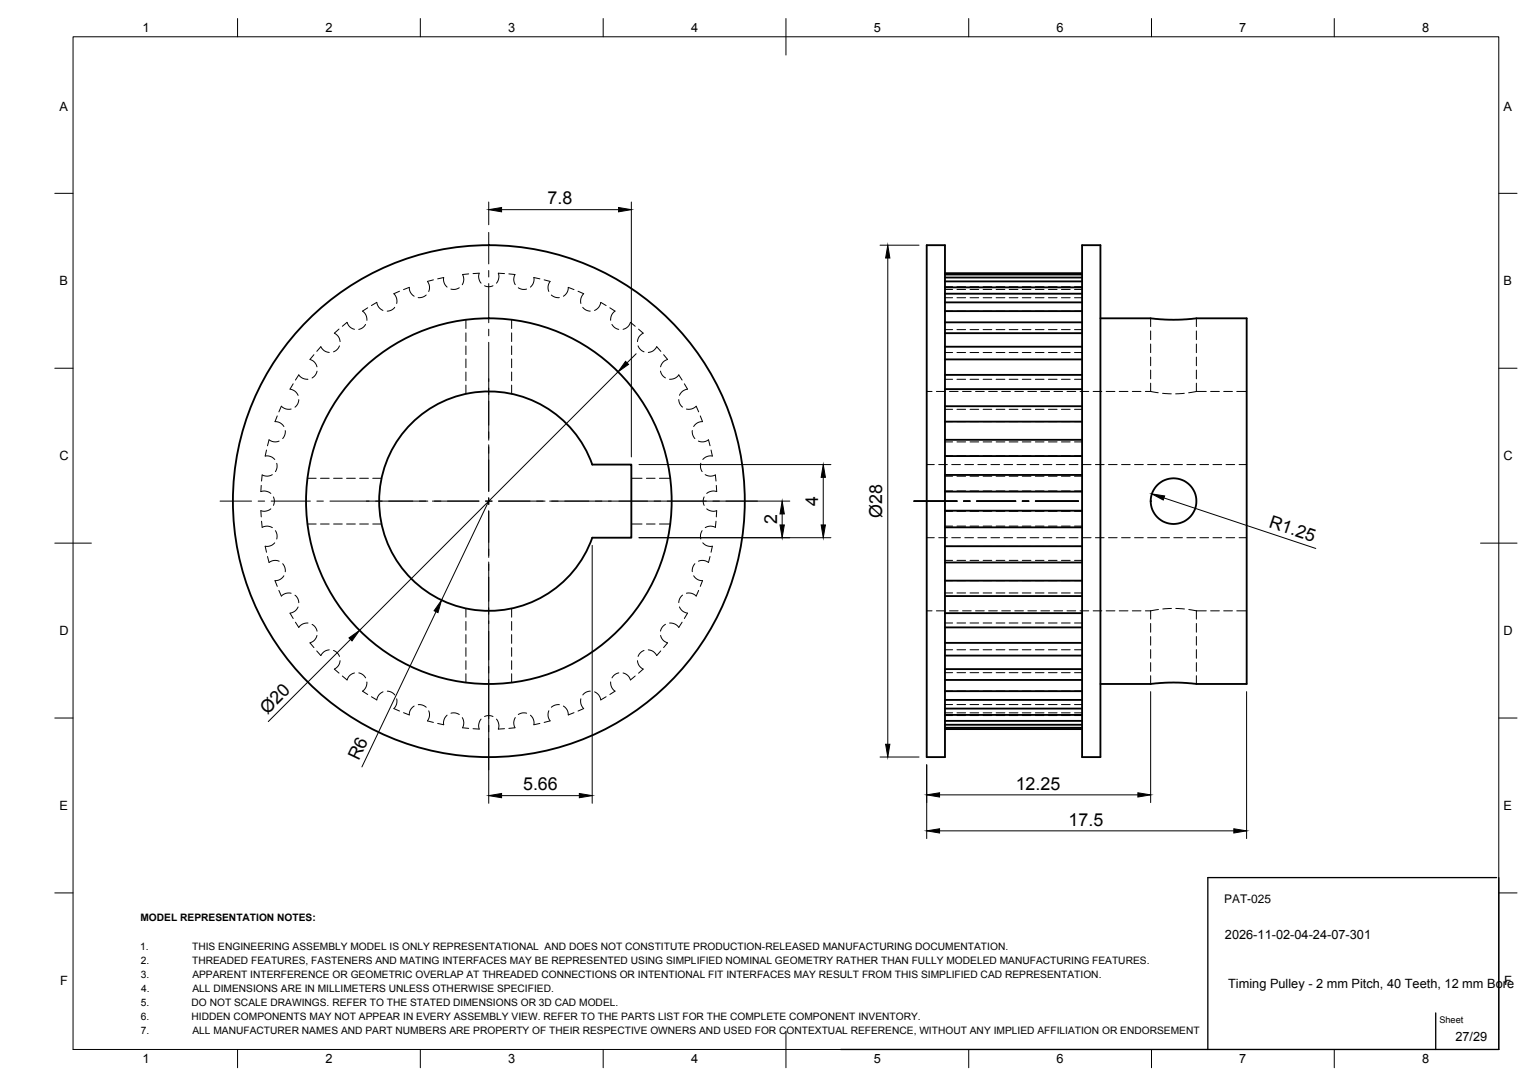
ISO-10303-21;
HEADER;
/* Generated by software containing ST-Developer
 * from STEP Tools, Inc. (www.steptools.com) 
 */

FILE_DESCRIPTION(
/* description */ ('Counter shaft with two pulleys and keyed hub'),
/* implementation_level */ '2;1');

FILE_NAME(
/* name */ 'Timing Pulley - 2 mm Pitch, 40 Teeth, 12 mm Bore.step',
/* time_stamp */ '2026-10-27T10:46:10-07:00',
/* author */ (''),
/* organization */ (''),
/* preprocessor_version */ 'ST-DEVELOPER v20.2',
/* originating_system */ 'Autodesk Translation Framework v15.17.0.0',
/* authorisation */ '');

FILE_SCHEMA (('AUTOMOTIVE_DESIGN { 1 0 10303 214 3 1 1 }'));
ENDSEC;

DATA;
#10=MECHANICAL_DESIGN_GEOMETRIC_PRESENTATION_REPRESENTATION('',(#311),#10821);
#220=B_SPLINE_CURVE_WITH_KNOTS('',3,(#9730,#9731,#9732,#9733,#9734,#9735,
#9736,#9737,#9738,#9739,#9740,#9741,#9742,#9743,#9744,#9745,#9746,#9747),
 .UNSPECIFIED.,.F.,.F.,(4,2,2,2,2,2,2,2,4),(0.,0.0472365751919841,0.0944731503839683,
0.14170659898184,0.188940047579712,0.236173496177583,0.283406944775455,
0.330643519967439,0.377880095159423),.UNSPECIFIED.);
#221=B_SPLINE_CURVE_WITH_KNOTS('',3,(#9748,#9749,#9750,#9751,#9752,#9753,
#9754,#9755,#9756,#9757,#9758,#9759,#9760,#9761,#9762,#9763,#9764,#9765),
 .UNSPECIFIED.,.F.,.F.,(4,2,2,2,2,2,2,2,4),(0.377880095159423,0.425116670351408,
0.472353245543392,0.519586694141263,0.566820142739135,0.614053591337007,
0.661287039934879,0.708523615126863,0.755760190318847),.UNSPECIFIED.);
#222=B_SPLINE_CURVE_WITH_KNOTS('',3,(#9768,#9769,#9770,#9771,#9772,#9773,
#9774,#9775,#9776,#9777,#9778,#9779,#9780,#9781,#9782,#9783,#9784,#9785),
 .UNSPECIFIED.,.F.,.F.,(4,2,2,2,2,2,2,2,4),(0.,0.0472365751919841,0.0944731503839682,
0.14170659898184,0.188940047579712,0.236173496177583,0.283406944775455,
0.330643519967439,0.377880095159423),.UNSPECIFIED.);
#223=B_SPLINE_CURVE_WITH_KNOTS('',3,(#9786,#9787,#9788,#9789,#9790,#9791,
#9792,#9793,#9794,#9795,#9796,#9797,#9798,#9799,#9800,#9801,#9802,#9803),
 .UNSPECIFIED.,.F.,.F.,(4,2,2,2,2,2,2,2,4),(0.377880095159423,0.425116670351408,
0.472353245543392,0.519586694141263,0.566820142739135,0.614053591337007,
0.661287039934879,0.708523615126863,0.755760190318847),.UNSPECIFIED.);
#224=B_SPLINE_CURVE_WITH_KNOTS('',3,(#9806,#9807,#9808,#9809,#9810,#9811,
#9812,#9813,#9814,#9815,#9816,#9817,#9818,#9819,#9820,#9821,#9822,#9823),
 .UNSPECIFIED.,.F.,.F.,(4,2,2,2,2,2,2,2,4),(0.,0.0472365751919841,0.0944731503839683,
0.14170659898184,0.188940047579712,0.236173496177583,0.283406944775455,
0.330643519967439,0.377880095159423),.UNSPECIFIED.);
#225=B_SPLINE_CURVE_WITH_KNOTS('',3,(#9824,#9825,#9826,#9827,#9828,#9829,
#9830,#9831,#9832,#9833,#9834,#9835,#9836,#9837,#9838,#9839,#9840,#9841),
 .UNSPECIFIED.,.F.,.F.,(4,2,2,2,2,2,2,2,4),(0.377880095159423,0.425116670351408,
0.472353245543392,0.519586694141263,0.566820142739135,0.614053591337007,
0.661287039934879,0.708523615126863,0.755760190318847),.UNSPECIFIED.);
#226=B_SPLINE_CURVE_WITH_KNOTS('',3,(#9845,#9846,#9847,#9848,#9849,#9850,
#9851,#9852,#9853,#9854),.UNSPECIFIED.,.F.,.F.,(4,2,2,2,4),(0.565665723963061,
0.61280433739166,0.659942950820258,0.70708195805217,0.754220965284082),
 .UNSPECIFIED.);
#227=B_SPLINE_CURVE_WITH_KNOTS('',3,(#9856,#9857,#9858,#9859,#9860,#9861,
#9862,#9863,#9864,#9865,#9866,#9867,#9868,#9869,#9870,#9871,#9872,#9873),
 .UNSPECIFIED.,.F.,.F.,(4,2,2,2,2,2,2,2,4),(0.18855524132102,0.235693854749619,
0.282832468178217,0.329971475410129,0.377110482642041,0.424249489873953,
0.471388497105864,0.518527110534463,0.565665723963061),.UNSPECIFIED.);
#228=B_SPLINE_CURVE_WITH_KNOTS('',3,(#9874,#9875,#9876,#9877,#9878,#9879,
#9880,#9881,#9882,#9883),.UNSPECIFIED.,.F.,.F.,(4,2,2,2,4),(0.754220965284082,
0.801359972515993,0.848498979747905,0.895637593176504,0.942776206605102),
 .UNSPECIFIED.);
#229=B_SPLINE_CURVE_WITH_KNOTS('',3,(#9889,#9890,#9891,#9892,#9893,#9894,
#9895,#9896,#9897,#9898),.UNSPECIFIED.,.F.,.F.,(4,2,2,2,4),(0.565665723963061,
0.61280433739166,0.659942950820258,0.70708195805217,0.754220965284082),
 .UNSPECIFIED.);
#230=B_SPLINE_CURVE_WITH_KNOTS('',3,(#9900,#9901,#9902,#9903,#9904,#9905,
#9906,#9907,#9908,#9909,#9910,#9911,#9912,#9913,#9914,#9915,#9916,#9917),
 .UNSPECIFIED.,.F.,.F.,(4,2,2,2,2,2,2,2,4),(0.18855524132102,0.235693854749619,
0.282832468178217,0.329971475410129,0.377110482642041,0.424249489873953,
0.471388497105864,0.518527110534463,0.565665723963061),.UNSPECIFIED.);
#231=B_SPLINE_CURVE_WITH_KNOTS('',3,(#9918,#9919,#9920,#9921,#9922,#9923,
#9924,#9925,#9926,#9927),.UNSPECIFIED.,.F.,.F.,(4,2,2,2,4),(0.754220965284082,
0.801359972515993,0.848498979747905,0.895637593176504,0.942776206605102),
 .UNSPECIFIED.);
#232=B_SPLINE_CURVE_WITH_KNOTS('',3,(#9937,#9938,#9939,#9940,#9941,#9942,
#9943,#9944,#9945,#9946,#9947,#9948,#9949,#9950,#9951,#9952,#9953,#9954),
 .UNSPECIFIED.,.F.,.F.,(4,2,2,2,2,2,2,2,4),(0.18855524132102,0.235693854749619,
0.282832468178217,0.329971475410129,0.377110482642041,0.424249489873953,
0.471388497105864,0.518527110534463,0.565665723963061),.UNSPECIFIED.);
#233=B_SPLINE_CURVE_WITH_KNOTS('',3,(#9956,#9957,#9958,#9959,#9960,#9961,
#9962,#9963,#9964,#9965),.UNSPECIFIED.,.F.,.F.,(4,2,2,2,4),(0.565665723963061,
0.61280433739166,0.659942950820258,0.70708195805217,0.754220965284082),
 .UNSPECIFIED.);
#234=B_SPLINE_CURVE_WITH_KNOTS('',3,(#9966,#9967,#9968,#9969,#9970,#9971,
#9972,#9973,#9974,#9975),.UNSPECIFIED.,.F.,.F.,(4,2,2,2,4),(0.754220965284082,
0.801359972515993,0.848498979747905,0.895637593176504,0.942776206605102),
 .UNSPECIFIED.);
#235=B_SPLINE_CURVE_WITH_KNOTS('',3,(#9978,#9979,#9980,#9981,#9982,#9983,
#9984,#9985,#9986,#9987,#9988,#9989,#9990,#9991,#9992,#9993,#9994,#9995),
 .UNSPECIFIED.,.F.,.F.,(4,2,2,2,2,2,2,2,4),(0.18855524132102,0.235693854749619,
0.282832468178217,0.329971475410129,0.377110482642041,0.424249489873953,
0.471388497105864,0.518527110534463,0.565665723963061),.UNSPECIFIED.);
#236=B_SPLINE_CURVE_WITH_KNOTS('',3,(#9997,#9998,#9999,#10000,#10001,#10002,
#10003,#10004,#10005,#10006),.UNSPECIFIED.,.F.,.F.,(4,2,2,2,4),(0.565665723963061,
0.61280433739166,0.659942950820258,0.70708195805217,0.754220965284082),
 .UNSPECIFIED.);
#237=B_SPLINE_CURVE_WITH_KNOTS('',3,(#10007,#10008,#10009,#10010,#10011,
#10012,#10013,#10014,#10015,#10016),.UNSPECIFIED.,.F.,.F.,(4,2,2,2,4),(0.754220965284082,
0.801359972515993,0.848498979747905,0.895637593176504,0.942776206605102),
 .UNSPECIFIED.);
#260=SHAPE_REPRESENTATION_RELATIONSHIP('SRR','None',#10948,#285);
#285=ADVANCED_BREP_SHAPE_REPRESENTATION('',(#336),#10816);
#311=STYLED_ITEM('',(#11128),#336);
#336=MANIFOLD_SOLID_BREP('Body1',#5595);
#417=FACE_BOUND('',#1150,.T.);
#418=FACE_BOUND('',#1153,.T.);
#419=FACE_BOUND('',#1155,.T.);
#420=FACE_BOUND('',#1156,.T.);
#421=FACE_BOUND('',#1157,.T.);
#422=FACE_BOUND('',#1161,.T.);
#423=FACE_BOUND('',#1162,.T.);
#424=FACE_BOUND('',#1163,.T.);
#425=FACE_BOUND('',#1167,.T.);
#426=FACE_BOUND('',#1169,.T.);
#427=FACE_BOUND('',#1172,.T.);
#428=FACE_BOUND('',#1174,.T.);
#540=PLANE('',#6208);
#541=PLANE('',#6209);
#542=PLANE('',#6211);
#543=PLANE('',#6212);
#544=PLANE('',#6224);
#545=PLANE('',#6225);
#546=PLANE('',#6309);
#547=PLANE('',#6310);
#757=FACE_OUTER_BOUND('',#1148,.T.);
#758=FACE_OUTER_BOUND('',#1149,.T.);
#759=FACE_OUTER_BOUND('',#1151,.T.);
#760=FACE_OUTER_BOUND('',#1152,.T.);
#761=FACE_OUTER_BOUND('',#1154,.T.);
#762=FACE_OUTER_BOUND('',#1158,.T.);
#763=FACE_OUTER_BOUND('',#1159,.T.);
#764=FACE_OUTER_BOUND('',#1160,.T.);
#765=FACE_OUTER_BOUND('',#1164,.T.);
#766=FACE_OUTER_BOUND('',#1165,.T.);
#767=FACE_OUTER_BOUND('',#1166,.T.);
#768=FACE_OUTER_BOUND('',#1168,.T.);
#769=FACE_OUTER_BOUND('',#1170,.T.);
#770=FACE_OUTER_BOUND('',#1171,.T.);
#771=FACE_OUTER_BOUND('',#1173,.T.);
#772=FACE_OUTER_BOUND('',#1175,.T.);
#773=FACE_OUTER_BOUND('',#1176,.T.);
#774=FACE_OUTER_BOUND('',#1177,.T.);
#775=FACE_OUTER_BOUND('',#1178,.T.);
#776=FACE_OUTER_BOUND('',#1179,.T.);
#777=FACE_OUTER_BOUND('',#1180,.T.);
#778=FACE_OUTER_BOUND('',#1181,.T.);
#779=FACE_OUTER_BOUND('',#1182,.T.);
#780=FACE_OUTER_BOUND('',#1183,.T.);
#781=FACE_OUTER_BOUND('',#1184,.T.);
#782=FACE_OUTER_BOUND('',#1185,.T.);
#783=FACE_OUTER_BOUND('',#1186,.T.);
#784=FACE_OUTER_BOUND('',#1187,.T.);
#785=FACE_OUTER_BOUND('',#1188,.T.);
#786=FACE_OUTER_BOUND('',#1189,.T.);
#787=FACE_OUTER_BOUND('',#1190,.T.);
#788=FACE_OUTER_BOUND('',#1191,.T.);
#789=FACE_OUTER_BOUND('',#1192,.T.);
#790=FACE_OUTER_BOUND('',#1193,.T.);
#791=FACE_OUTER_BOUND('',#1194,.T.);
#792=FACE_OUTER_BOUND('',#1195,.T.);
#793=FACE_OUTER_BOUND('',#1196,.T.);
#794=FACE_OUTER_BOUND('',#1197,.T.);
#795=FACE_OUTER_BOUND('',#1198,.T.);
#796=FACE_OUTER_BOUND('',#1199,.T.);
#797=FACE_OUTER_BOUND('',#1200,.T.);
#798=FACE_OUTER_BOUND('',#1201,.T.);
#799=FACE_OUTER_BOUND('',#1202,.T.);
#800=FACE_OUTER_BOUND('',#1203,.T.);
#801=FACE_OUTER_BOUND('',#1204,.T.);
#802=FACE_OUTER_BOUND('',#1205,.T.);
#803=FACE_OUTER_BOUND('',#1206,.T.);
#804=FACE_OUTER_BOUND('',#1207,.T.);
#805=FACE_OUTER_BOUND('',#1208,.T.);
#806=FACE_OUTER_BOUND('',#1209,.T.);
#807=FACE_OUTER_BOUND('',#1210,.T.);
#808=FACE_OUTER_BOUND('',#1211,.T.);
#809=FACE_OUTER_BOUND('',#1212,.T.);
#810=FACE_OUTER_BOUND('',#1213,.T.);
#811=FACE_OUTER_BOUND('',#1214,.T.);
#812=FACE_OUTER_BOUND('',#1215,.T.);
#813=FACE_OUTER_BOUND('',#1216,.T.);
#814=FACE_OUTER_BOUND('',#1217,.T.);
#815=FACE_OUTER_BOUND('',#1218,.T.);
#816=FACE_OUTER_BOUND('',#1219,.T.);
#817=FACE_OUTER_BOUND('',#1220,.T.);
#818=FACE_OUTER_BOUND('',#1221,.T.);
#819=FACE_OUTER_BOUND('',#1222,.T.);
#820=FACE_OUTER_BOUND('',#1223,.T.);
#821=FACE_OUTER_BOUND('',#1224,.T.);
#822=FACE_OUTER_BOUND('',#1225,.T.);
#823=FACE_OUTER_BOUND('',#1226,.T.);
#824=FACE_OUTER_BOUND('',#1227,.T.);
#825=FACE_OUTER_BOUND('',#1228,.T.);
#826=FACE_OUTER_BOUND('',#1229,.T.);
#827=FACE_OUTER_BOUND('',#1230,.T.);
#828=FACE_OUTER_BOUND('',#1231,.T.);
#829=FACE_OUTER_BOUND('',#1232,.T.);
#830=FACE_OUTER_BOUND('',#1233,.T.);
#831=FACE_OUTER_BOUND('',#1234,.T.);
#832=FACE_OUTER_BOUND('',#1235,.T.);
#833=FACE_OUTER_BOUND('',#1236,.T.);
#834=FACE_OUTER_BOUND('',#1237,.T.);
#835=FACE_OUTER_BOUND('',#1238,.T.);
#836=FACE_OUTER_BOUND('',#1239,.T.);
#837=FACE_OUTER_BOUND('',#1240,.T.);
#838=FACE_OUTER_BOUND('',#1241,.T.);
#839=FACE_OUTER_BOUND('',#1242,.T.);
#840=FACE_OUTER_BOUND('',#1243,.T.);
#841=FACE_OUTER_BOUND('',#1244,.T.);
#842=FACE_OUTER_BOUND('',#1245,.T.);
#843=FACE_OUTER_BOUND('',#1246,.T.);
#844=FACE_OUTER_BOUND('',#1247,.T.);
#845=FACE_OUTER_BOUND('',#1248,.T.);
#846=FACE_OUTER_BOUND('',#1249,.T.);
#847=FACE_OUTER_BOUND('',#1250,.T.);
#848=FACE_OUTER_BOUND('',#1251,.T.);
#849=FACE_OUTER_BOUND('',#1252,.T.);
#850=FACE_OUTER_BOUND('',#1253,.T.);
#851=FACE_OUTER_BOUND('',#1254,.T.);
#852=FACE_OUTER_BOUND('',#1255,.T.);
#1148=EDGE_LOOP('',(#4333,#4334,#4335,#4336));
#1149=EDGE_LOOP('',(#4337,#4338,#4339,#4340));
#1150=EDGE_LOOP('',(#4341));
#1151=EDGE_LOOP('',(#4342,#4343,#4344,#4345));
#1152=EDGE_LOOP('',(#4346));
#1153=EDGE_LOOP('',(#4347,#4348,#4349,#4350));
#1154=EDGE_LOOP('',(#4351,#4352,#4353,#4354));
#1155=EDGE_LOOP('',(#4355,#4356));
#1156=EDGE_LOOP('',(#4357,#4358));
#1157=EDGE_LOOP('',(#4359,#4360));
#1158=EDGE_LOOP('',(#4361,#4362,#4363,#4364,#4365,#4366,#4367));
#1159=EDGE_LOOP('',(#4368,#4369,#4370,#4371,#4372,#4373,#4374));
#1160=EDGE_LOOP('',(#4375,#4376,#4377,#4378,#4379,#4380,#4381,#4382,#4383));
#1161=EDGE_LOOP('',(#4384,#4385,#4386));
#1162=EDGE_LOOP('',(#4387,#4388,#4389));
#1163=EDGE_LOOP('',(#4390,#4391,#4392));
#1164=EDGE_LOOP('',(#4393,#4394,#4395,#4396,#4397,#4398));
#1165=EDGE_LOOP('',(#4399,#4400,#4401,#4402,#4403,#4404,#4405));
#1166=EDGE_LOOP('',(#4406));
#1167=EDGE_LOOP('',(#4407,#4408,#4409,#4410));
#1168=EDGE_LOOP('',(#4411));
#1169=EDGE_LOOP('',(#4412,#4413,#4414,#4415,#4416,#4417,#4418,#4419,#4420,
#4421,#4422,#4423,#4424,#4425,#4426,#4427,#4428,#4429,#4430,#4431,#4432,
#4433,#4434,#4435,#4436,#4437,#4438,#4439,#4440,#4441,#4442,#4443,#4444,
#4445,#4446,#4447,#4448,#4449,#4450,#4451,#4452,#4453,#4454,#4455,#4456,
#4457,#4458,#4459,#4460,#4461,#4462,#4463,#4464,#4465,#4466,#4467,#4468,
#4469,#4470,#4471,#4472,#4473,#4474,#4475,#4476,#4477,#4478,#4479,#4480,
#4481,#4482,#4483,#4484,#4485,#4486,#4487,#4488,#4489,#4490,#4491));
#1170=EDGE_LOOP('',(#4492,#4493,#4494,#4495));
#1171=EDGE_LOOP('',(#4496));
#1172=EDGE_LOOP('',(#4497));
#1173=EDGE_LOOP('',(#4498));
#1174=EDGE_LOOP('',(#4499,#4500,#4501,#4502,#4503,#4504,#4505,#4506,#4507,
#4508,#4509,#4510,#4511,#4512,#4513,#4514,#4515,#4516,#4517,#4518,#4519,
#4520,#4521,#4522,#4523,#4524,#4525,#4526,#4527,#4528,#4529,#4530,#4531,
#4532,#4533,#4534,#4535,#4536,#4537,#4538,#4539,#4540,#4541,#4542,#4543,
#4544,#4545,#4546,#4547,#4548,#4549,#4550,#4551,#4552,#4553,#4554,#4555,
#4556,#4557,#4558,#4559,#4560,#4561,#4562,#4563,#4564,#4565,#4566,#4567,
#4568,#4569,#4570,#4571,#4572,#4573,#4574,#4575,#4576,#4577,#4578));
#1175=EDGE_LOOP('',(#4579,#4580,#4581,#4582));
#1176=EDGE_LOOP('',(#4583,#4584,#4585,#4586));
#1177=EDGE_LOOP('',(#4587,#4588,#4589,#4590));
#1178=EDGE_LOOP('',(#4591,#4592,#4593,#4594));
#1179=EDGE_LOOP('',(#4595,#4596,#4597,#4598));
#1180=EDGE_LOOP('',(#4599,#4600,#4601,#4602));
#1181=EDGE_LOOP('',(#4603,#4604,#4605,#4606));
#1182=EDGE_LOOP('',(#4607,#4608,#4609,#4610));
#1183=EDGE_LOOP('',(#4611,#4612,#4613,#4614));
#1184=EDGE_LOOP('',(#4615,#4616,#4617,#4618));
#1185=EDGE_LOOP('',(#4619,#4620,#4621,#4622));
#1186=EDGE_LOOP('',(#4623,#4624,#4625,#4626));
#1187=EDGE_LOOP('',(#4627,#4628,#4629,#4630));
#1188=EDGE_LOOP('',(#4631,#4632,#4633,#4634));
#1189=EDGE_LOOP('',(#4635,#4636,#4637,#4638));
#1190=EDGE_LOOP('',(#4639,#4640,#4641,#4642));
#1191=EDGE_LOOP('',(#4643,#4644,#4645,#4646));
#1192=EDGE_LOOP('',(#4647,#4648,#4649,#4650));
#1193=EDGE_LOOP('',(#4651,#4652,#4653,#4654));
#1194=EDGE_LOOP('',(#4655,#4656,#4657,#4658));
#1195=EDGE_LOOP('',(#4659,#4660,#4661,#4662));
#1196=EDGE_LOOP('',(#4663,#4664,#4665,#4666));
#1197=EDGE_LOOP('',(#4667,#4668,#4669,#4670));
#1198=EDGE_LOOP('',(#4671,#4672,#4673,#4674));
#1199=EDGE_LOOP('',(#4675,#4676,#4677,#4678));
#1200=EDGE_LOOP('',(#4679,#4680,#4681,#4682));
#1201=EDGE_LOOP('',(#4683,#4684,#4685,#4686));
#1202=EDGE_LOOP('',(#4687,#4688,#4689,#4690));
#1203=EDGE_LOOP('',(#4691,#4692,#4693,#4694));
#1204=EDGE_LOOP('',(#4695,#4696,#4697,#4698));
#1205=EDGE_LOOP('',(#4699,#4700,#4701,#4702));
#1206=EDGE_LOOP('',(#4703,#4704,#4705,#4706));
#1207=EDGE_LOOP('',(#4707,#4708,#4709,#4710));
#1208=EDGE_LOOP('',(#4711,#4712,#4713,#4714));
#1209=EDGE_LOOP('',(#4715,#4716,#4717,#4718));
#1210=EDGE_LOOP('',(#4719,#4720,#4721,#4722));
#1211=EDGE_LOOP('',(#4723,#4724,#4725,#4726));
#1212=EDGE_LOOP('',(#4727,#4728,#4729,#4730));
#1213=EDGE_LOOP('',(#4731,#4732,#4733,#4734));
#1214=EDGE_LOOP('',(#4735,#4736,#4737,#4738));
#1215=EDGE_LOOP('',(#4739,#4740,#4741,#4742));
#1216=EDGE_LOOP('',(#4743,#4744,#4745,#4746));
#1217=EDGE_LOOP('',(#4747,#4748,#4749,#4750));
#1218=EDGE_LOOP('',(#4751,#4752,#4753,#4754));
#1219=EDGE_LOOP('',(#4755,#4756,#4757,#4758));
#1220=EDGE_LOOP('',(#4759,#4760,#4761,#4762));
#1221=EDGE_LOOP('',(#4763,#4764,#4765,#4766));
#1222=EDGE_LOOP('',(#4767,#4768,#4769,#4770));
#1223=EDGE_LOOP('',(#4771,#4772,#4773,#4774));
#1224=EDGE_LOOP('',(#4775,#4776,#4777,#4778));
#1225=EDGE_LOOP('',(#4779,#4780,#4781,#4782));
#1226=EDGE_LOOP('',(#4783,#4784,#4785,#4786));
#1227=EDGE_LOOP('',(#4787,#4788,#4789,#4790));
#1228=EDGE_LOOP('',(#4791,#4792,#4793,#4794));
#1229=EDGE_LOOP('',(#4795,#4796,#4797,#4798));
#1230=EDGE_LOOP('',(#4799,#4800,#4801,#4802));
#1231=EDGE_LOOP('',(#4803,#4804,#4805,#4806));
#1232=EDGE_LOOP('',(#4807,#4808,#4809,#4810));
#1233=EDGE_LOOP('',(#4811,#4812,#4813,#4814));
#1234=EDGE_LOOP('',(#4815,#4816,#4817,#4818));
#1235=EDGE_LOOP('',(#4819,#4820,#4821,#4822));
#1236=EDGE_LOOP('',(#4823,#4824,#4825,#4826));
#1237=EDGE_LOOP('',(#4827,#4828,#4829,#4830));
#1238=EDGE_LOOP('',(#4831,#4832,#4833,#4834));
#1239=EDGE_LOOP('',(#4835,#4836,#4837,#4838));
#1240=EDGE_LOOP('',(#4839,#4840,#4841,#4842));
#1241=EDGE_LOOP('',(#4843,#4844,#4845,#4846));
#1242=EDGE_LOOP('',(#4847,#4848,#4849,#4850));
#1243=EDGE_LOOP('',(#4851,#4852,#4853,#4854));
#1244=EDGE_LOOP('',(#4855,#4856,#4857,#4858));
#1245=EDGE_LOOP('',(#4859,#4860,#4861,#4862));
#1246=EDGE_LOOP('',(#4863,#4864,#4865,#4866));
#1247=EDGE_LOOP('',(#4867,#4868,#4869,#4870));
#1248=EDGE_LOOP('',(#4871,#4872,#4873,#4874));
#1249=EDGE_LOOP('',(#4875,#4876,#4877,#4878));
#1250=EDGE_LOOP('',(#4879,#4880,#4881,#4882));
#1251=EDGE_LOOP('',(#4883,#4884,#4885,#4886));
#1252=EDGE_LOOP('',(#4887,#4888,#4889,#4890));
#1253=EDGE_LOOP('',(#4891,#4892,#4893,#4894));
#1254=EDGE_LOOP('',(#4895,#4896,#4897,#4898));
#1255=EDGE_LOOP('',(#4899,#4900,#4901,#4902));
#1505=LINE('',#9702,#1894);
#1506=LINE('',#9704,#1895);
#1507=LINE('',#9706,#1896);
#1508=LINE('',#9707,#1897);
#1509=LINE('',#9710,#1898);
#1510=LINE('',#9712,#1899);
#1511=LINE('',#9713,#1900);
#1512=LINE('',#9718,#1901);
#1513=LINE('',#9720,#1902);
#1514=LINE('',#9721,#1903);
#1515=LINE('',#9884,#1904);
#1516=LINE('',#9887,#1905);
#1517=LINE('',#9931,#1906);
#1518=LINE('',#9933,#1907);
#1519=LINE('',#10018,#1908);
#1520=LINE('',#10020,#1909);
#1521=LINE('',#10188,#1910);
#1522=LINE('',#10354,#1911);
#1523=LINE('',#10356,#1912);
#1524=LINE('',#10357,#1913);
#1525=LINE('',#10359,#1914);
#1526=LINE('',#10361,#1915);
#1527=LINE('',#10363,#1916);
#1528=LINE('',#10365,#1917);
#1529=LINE('',#10367,#1918);
#1530=LINE('',#10369,#1919);
#1531=LINE('',#10371,#1920);
#1532=LINE('',#10373,#1921);
#1533=LINE('',#10375,#1922);
#1534=LINE('',#10377,#1923);
#1535=LINE('',#10379,#1924);
#1536=LINE('',#10381,#1925);
#1537=LINE('',#10383,#1926);
#1538=LINE('',#10385,#1927);
#1539=LINE('',#10387,#1928);
#1540=LINE('',#10389,#1929);
#1541=LINE('',#10391,#1930);
#1542=LINE('',#10393,#1931);
#1543=LINE('',#10395,#1932);
#1544=LINE('',#10397,#1933);
#1545=LINE('',#10399,#1934);
#1546=LINE('',#10401,#1935);
#1547=LINE('',#10403,#1936);
#1548=LINE('',#10405,#1937);
#1549=LINE('',#10407,#1938);
#1550=LINE('',#10409,#1939);
#1551=LINE('',#10411,#1940);
#1552=LINE('',#10413,#1941);
#1553=LINE('',#10415,#1942);
#1554=LINE('',#10417,#1943);
#1555=LINE('',#10419,#1944);
#1556=LINE('',#10421,#1945);
#1557=LINE('',#10423,#1946);
#1558=LINE('',#10425,#1947);
#1559=LINE('',#10427,#1948);
#1560=LINE('',#10429,#1949);
#1561=LINE('',#10431,#1950);
#1562=LINE('',#10433,#1951);
#1563=LINE('',#10435,#1952);
#1564=LINE('',#10437,#1953);
#1565=LINE('',#10439,#1954);
#1566=LINE('',#10441,#1955);
#1567=LINE('',#10443,#1956);
#1568=LINE('',#10445,#1957);
#1569=LINE('',#10447,#1958);
#1570=LINE('',#10449,#1959);
#1571=LINE('',#10451,#1960);
#1572=LINE('',#10453,#1961);
#1573=LINE('',#10455,#1962);
#1574=LINE('',#10457,#1963);
#1575=LINE('',#10459,#1964);
#1576=LINE('',#10461,#1965);
#1577=LINE('',#10463,#1966);
#1578=LINE('',#10465,#1967);
#1579=LINE('',#10467,#1968);
#1580=LINE('',#10469,#1969);
#1581=LINE('',#10471,#1970);
#1582=LINE('',#10473,#1971);
#1583=LINE('',#10475,#1972);
#1584=LINE('',#10477,#1973);
#1585=LINE('',#10479,#1974);
#1586=LINE('',#10481,#1975);
#1587=LINE('',#10483,#1976);
#1588=LINE('',#10485,#1977);
#1589=LINE('',#10487,#1978);
#1590=LINE('',#10489,#1979);
#1591=LINE('',#10491,#1980);
#1592=LINE('',#10493,#1981);
#1593=LINE('',#10495,#1982);
#1594=LINE('',#10497,#1983);
#1595=LINE('',#10499,#1984);
#1596=LINE('',#10501,#1985);
#1597=LINE('',#10503,#1986);
#1598=LINE('',#10505,#1987);
#1599=LINE('',#10507,#1988);
#1600=LINE('',#10509,#1989);
#1601=LINE('',#10511,#1990);
#1602=LINE('',#10513,#1991);
#1894=VECTOR('',#7421,1.);
#1895=VECTOR('',#7422,1.);
#1896=VECTOR('',#7423,1.);
#1897=VECTOR('',#7424,1.);
#1898=VECTOR('',#7427,1.);
#1899=VECTOR('',#7428,1.);
#1900=VECTOR('',#7429,1.);
#1901=VECTOR('',#7434,1.);
#1902=VECTOR('',#7435,1.);
#1903=VECTOR('',#7436,1.);
#1904=VECTOR('',#7449,0.125);
#1905=VECTOR('',#7452,0.125);
#1906=VECTOR('',#7457,1.);
#1907=VECTOR('',#7458,1.);
#1908=VECTOR('',#7463,0.125);
#1909=VECTOR('',#7466,0.125);
#1910=VECTOR('',#7637,1.4);
#1911=VECTOR('',#7806,1.4);
#1912=VECTOR('',#7809,1.);
#1913=VECTOR('',#7810,1.);
#1914=VECTOR('',#7813,1.);
#1915=VECTOR('',#7816,1.);
#1916=VECTOR('',#7819,1.);
#1917=VECTOR('',#7822,1.);
#1918=VECTOR('',#7825,1.);
#1919=VECTOR('',#7828,1.);
#1920=VECTOR('',#7831,1.);
#1921=VECTOR('',#7834,1.);
#1922=VECTOR('',#7837,1.);
#1923=VECTOR('',#7840,1.);
#1924=VECTOR('',#7843,1.);
#1925=VECTOR('',#7846,1.);
#1926=VECTOR('',#7849,1.);
#1927=VECTOR('',#7852,1.);
#1928=VECTOR('',#7855,1.);
#1929=VECTOR('',#7858,1.);
#1930=VECTOR('',#7861,1.);
#1931=VECTOR('',#7864,1.);
#1932=VECTOR('',#7867,1.);
#1933=VECTOR('',#7870,1.);
#1934=VECTOR('',#7873,1.);
#1935=VECTOR('',#7876,1.);
#1936=VECTOR('',#7879,1.);
#1937=VECTOR('',#7882,1.);
#1938=VECTOR('',#7885,1.);
#1939=VECTOR('',#7888,1.);
#1940=VECTOR('',#7891,1.);
#1941=VECTOR('',#7894,1.);
#1942=VECTOR('',#7897,1.);
#1943=VECTOR('',#7900,1.);
#1944=VECTOR('',#7903,1.);
#1945=VECTOR('',#7906,1.);
#1946=VECTOR('',#7909,1.);
#1947=VECTOR('',#7912,1.);
#1948=VECTOR('',#7915,1.);
#1949=VECTOR('',#7918,1.);
#1950=VECTOR('',#7921,1.);
#1951=VECTOR('',#7924,1.);
#1952=VECTOR('',#7927,1.);
#1953=VECTOR('',#7930,1.);
#1954=VECTOR('',#7933,1.);
#1955=VECTOR('',#7936,1.);
#1956=VECTOR('',#7939,1.);
#1957=VECTOR('',#7942,1.);
#1958=VECTOR('',#7945,1.);
#1959=VECTOR('',#7948,1.);
#1960=VECTOR('',#7951,1.);
#1961=VECTOR('',#7954,1.);
#1962=VECTOR('',#7957,1.);
#1963=VECTOR('',#7960,1.);
#1964=VECTOR('',#7963,1.);
#1965=VECTOR('',#7966,1.);
#1966=VECTOR('',#7969,1.);
#1967=VECTOR('',#7972,1.);
#1968=VECTOR('',#7975,1.);
#1969=VECTOR('',#7978,1.);
#1970=VECTOR('',#7981,1.);
#1971=VECTOR('',#7984,1.);
#1972=VECTOR('',#7987,1.);
#1973=VECTOR('',#7990,1.);
#1974=VECTOR('',#7993,1.);
#1975=VECTOR('',#7996,1.);
#1976=VECTOR('',#7999,1.);
#1977=VECTOR('',#8002,1.);
#1978=VECTOR('',#8005,1.);
#1979=VECTOR('',#8008,1.);
#1980=VECTOR('',#8011,1.);
#1981=VECTOR('',#8014,1.);
#1982=VECTOR('',#8017,1.);
#1983=VECTOR('',#8020,1.);
#1984=VECTOR('',#8023,1.);
#1985=VECTOR('',#8026,1.);
#1986=VECTOR('',#8029,1.);
#1987=VECTOR('',#8032,1.);
#1988=VECTOR('',#8035,1.);
#1989=VECTOR('',#8038,1.);
#1990=VECTOR('',#8041,1.);
#1991=VECTOR('',#8044,1.);
#2203=CIRCLE('',#6210,0.125);
#2204=CIRCLE('',#6213,1.4);
#2205=CIRCLE('',#6214,0.6);
#2206=CIRCLE('',#6216,0.6);
#2207=CIRCLE('',#6220,1.);
#2208=CIRCLE('',#6221,1.);
#2209=CIRCLE('',#6226,1.4);
#2210=CIRCLE('',#6227,0.0555000000000001);
#2211=CIRCLE('',#6228,1.24783954473516);
#2212=CIRCLE('',#6229,0.0555000000000001);
#2213=CIRCLE('',#6230,1.24783954473516);
#2214=CIRCLE('',#6231,0.0555000000000001);
#2215=CIRCLE('',#6232,1.24783954473516);
#2216=CIRCLE('',#6233,0.0555000000000001);
#2217=CIRCLE('',#6234,1.24783954473516);
#2218=CIRCLE('',#6235,0.0555000000000001);
#2219=CIRCLE('',#6236,1.24783954473516);
#2220=CIRCLE('',#6237,0.0555000000000001);
#2221=CIRCLE('',#6238,1.24783954473516);
#2222=CIRCLE('',#6239,0.0555000000000001);
#2223=CIRCLE('',#6240,1.24783954473516);
#2224=CIRCLE('',#6241,0.0555000000000001);
#2225=CIRCLE('',#6242,1.24783954473516);
#2226=CIRCLE('',#6243,0.0555000000000001);
#2227=CIRCLE('',#6244,1.24783954473516);
#2228=CIRCLE('',#6245,0.0555000000000001);
#2229=CIRCLE('',#6246,1.24783954473516);
#2230=CIRCLE('',#6247,0.0555000000000001);
#2231=CIRCLE('',#6248,1.24783954473516);
#2232=CIRCLE('',#6249,0.0555000000000001);
#2233=CIRCLE('',#6250,1.24783954473516);
#2234=CIRCLE('',#6251,0.0555000000000001);
#2235=CIRCLE('',#6252,1.24783954473516);
#2236=CIRCLE('',#6253,0.0555000000000001);
#2237=CIRCLE('',#6254,1.24783954473516);
#2238=CIRCLE('',#6255,0.0555000000000001);
#2239=CIRCLE('',#6256,1.24783954473516);
#2240=CIRCLE('',#6257,0.0555000000000001);
#2241=CIRCLE('',#6258,1.24783954473516);
#2242=CIRCLE('',#6259,0.0555000000000001);
#2243=CIRCLE('',#6260,1.24783954473516);
#2244=CIRCLE('',#6261,0.0555000000000001);
#2245=CIRCLE('',#6262,1.24783954473516);
#2246=CIRCLE('',#6263,0.0555000000000001);
#2247=CIRCLE('',#6264,1.24783954473516);
#2248=CIRCLE('',#6265,0.0555000000000001);
#2249=CIRCLE('',#6266,1.24783954473516);
#2250=CIRCLE('',#6267,0.0555000000000001);
#2251=CIRCLE('',#6268,1.24783954473516);
#2252=CIRCLE('',#6269,0.0555000000000001);
#2253=CIRCLE('',#6270,1.24783954473516);
#2254=CIRCLE('',#6271,0.0555000000000001);
#2255=CIRCLE('',#6272,1.24783954473516);
#2256=CIRCLE('',#6273,0.0555000000000001);
#2257=CIRCLE('',#6274,1.24783954473516);
#2258=CIRCLE('',#6275,0.0555000000000001);
#2259=CIRCLE('',#6276,1.24783954473516);
#2260=CIRCLE('',#6277,0.0555000000000001);
#2261=CIRCLE('',#6278,1.24783954473516);
#2262=CIRCLE('',#6279,0.0555000000000001);
#2263=CIRCLE('',#6280,1.24783954473516);
#2264=CIRCLE('',#6281,0.0555000000000001);
#2265=CIRCLE('',#6282,1.24783954473516);
#2266=CIRCLE('',#6283,0.0555000000000001);
#2267=CIRCLE('',#6284,1.24783954473516);
#2268=CIRCLE('',#6285,0.0555000000000001);
#2269=CIRCLE('',#6286,1.24783954473516);
#2270=CIRCLE('',#6287,0.0555000000000001);
#2271=CIRCLE('',#6288,1.24783954473516);
#2272=CIRCLE('',#6289,0.0555000000000001);
#2273=CIRCLE('',#6290,1.24783954473516);
#2274=CIRCLE('',#6291,0.0555000000000001);
#2275=CIRCLE('',#6292,1.24783954473516);
#2276=CIRCLE('',#6293,0.0555000000000001);
#2277=CIRCLE('',#6294,1.24783954473516);
#2278=CIRCLE('',#6295,0.0555000000000001);
#2279=CIRCLE('',#6296,1.24783954473516);
#2280=CIRCLE('',#6297,0.0555000000000001);
#2281=CIRCLE('',#6298,1.24783954473516);
#2282=CIRCLE('',#6299,0.0555000000000001);
#2283=CIRCLE('',#6300,1.24783954473516);
#2284=CIRCLE('',#6301,0.0555000000000001);
#2285=CIRCLE('',#6302,1.24783954473516);
#2286=CIRCLE('',#6303,0.0555000000000001);
#2287=CIRCLE('',#6304,1.24783954473516);
#2288=CIRCLE('',#6305,0.0555000000000001);
#2289=CIRCLE('',#6306,1.24783954473516);
#2290=CIRCLE('',#6308,1.4);
#2291=CIRCLE('',#6311,1.4);
#2292=CIRCLE('',#6312,0.0555000000000001);
#2293=CIRCLE('',#6313,1.24783954473516);
#2294=CIRCLE('',#6314,0.0555000000000001);
#2295=CIRCLE('',#6315,1.24783954473516);
#2296=CIRCLE('',#6316,0.0555000000000001);
#2297=CIRCLE('',#6317,1.24783954473516);
#2298=CIRCLE('',#6318,0.0555000000000001);
#2299=CIRCLE('',#6319,1.24783954473516);
#2300=CIRCLE('',#6320,0.0555000000000001);
#2301=CIRCLE('',#6321,1.24783954473516);
#2302=CIRCLE('',#6322,0.0555000000000001);
#2303=CIRCLE('',#6323,1.24783954473516);
#2304=CIRCLE('',#6324,0.0555000000000001);
#2305=CIRCLE('',#6325,1.24783954473516);
#2306=CIRCLE('',#6326,0.0555000000000001);
#2307=CIRCLE('',#6327,1.24783954473516);
#2308=CIRCLE('',#6328,0.0555000000000001);
#2309=CIRCLE('',#6329,1.24783954473516);
#2310=CIRCLE('',#6330,0.0555000000000001);
#2311=CIRCLE('',#6331,1.24783954473516);
#2312=CIRCLE('',#6332,0.0555000000000001);
#2313=CIRCLE('',#6333,1.24783954473516);
#2314=CIRCLE('',#6334,0.0555000000000001);
#2315=CIRCLE('',#6335,1.24783954473516);
#2316=CIRCLE('',#6336,0.0555000000000001);
#2317=CIRCLE('',#6337,1.24783954473516);
#2318=CIRCLE('',#6338,0.0555000000000001);
#2319=CIRCLE('',#6339,1.24783954473516);
#2320=CIRCLE('',#6340,0.0555000000000001);
#2321=CIRCLE('',#6341,1.24783954473516);
#2322=CIRCLE('',#6342,0.0555000000000001);
#2323=CIRCLE('',#6343,1.24783954473516);
#2324=CIRCLE('',#6344,0.0555000000000001);
#2325=CIRCLE('',#6345,1.24783954473516);
#2326=CIRCLE('',#6346,0.0555000000000001);
#2327=CIRCLE('',#6347,1.24783954473516);
#2328=CIRCLE('',#6348,0.0555000000000001);
#2329=CIRCLE('',#6349,1.24783954473516);
#2330=CIRCLE('',#6350,0.0555000000000001);
#2331=CIRCLE('',#6351,1.24783954473516);
#2332=CIRCLE('',#6352,0.0555000000000001);
#2333=CIRCLE('',#6353,1.24783954473516);
#2334=CIRCLE('',#6354,0.0555000000000001);
#2335=CIRCLE('',#6355,1.24783954473516);
#2336=CIRCLE('',#6356,0.0555000000000001);
#2337=CIRCLE('',#6357,1.24783954473516);
#2338=CIRCLE('',#6358,0.0555000000000001);
#2339=CIRCLE('',#6359,1.24783954473516);
#2340=CIRCLE('',#6360,0.0555000000000001);
#2341=CIRCLE('',#6361,1.24783954473516);
#2342=CIRCLE('',#6362,0.0555000000000001);
#2343=CIRCLE('',#6363,1.24783954473516);
#2344=CIRCLE('',#6364,0.0555000000000001);
#2345=CIRCLE('',#6365,1.24783954473516);
#2346=CIRCLE('',#6366,0.0555000000000001);
#2347=CIRCLE('',#6367,1.24783954473516);
#2348=CIRCLE('',#6368,0.0555000000000001);
#2349=CIRCLE('',#6369,1.24783954473516);
#2350=CIRCLE('',#6370,0.0555000000000001);
#2351=CIRCLE('',#6371,1.24783954473516);
#2352=CIRCLE('',#6372,0.0555000000000001);
#2353=CIRCLE('',#6373,1.24783954473516);
#2354=CIRCLE('',#6374,0.0555000000000001);
#2355=CIRCLE('',#6375,1.24783954473516);
#2356=CIRCLE('',#6376,0.0555000000000001);
#2357=CIRCLE('',#6377,1.24783954473516);
#2358=CIRCLE('',#6378,0.0555000000000001);
#2359=CIRCLE('',#6379,1.24783954473516);
#2360=CIRCLE('',#6380,0.0555000000000001);
#2361=CIRCLE('',#6381,1.24783954473516);
#2362=CIRCLE('',#6382,0.0555000000000001);
#2363=CIRCLE('',#6383,1.24783954473516);
#2364=CIRCLE('',#6384,0.0555000000000001);
#2365=CIRCLE('',#6385,1.24783954473516);
#2366=CIRCLE('',#6386,0.0555000000000001);
#2367=CIRCLE('',#6387,1.24783954473516);
#2368=CIRCLE('',#6388,0.0555000000000001);
#2369=CIRCLE('',#6389,1.24783954473516);
#2370=CIRCLE('',#6390,0.0555000000000001);
#2371=CIRCLE('',#6391,1.24783954473516);
#2626=VERTEX_POINT('',#9700);
#2627=VERTEX_POINT('',#9701);
#2628=VERTEX_POINT('',#9703);
#2629=VERTEX_POINT('',#9705);
#2630=VERTEX_POINT('',#9709);
#2631=VERTEX_POINT('',#9711);
#2632=VERTEX_POINT('',#9714);
#2633=VERTEX_POINT('',#9717);
#2634=VERTEX_POINT('',#9719);
#2635=VERTEX_POINT('',#9723);
#2636=VERTEX_POINT('',#9728);
#2637=VERTEX_POINT('',#9729);
#2638=VERTEX_POINT('',#9766);
#2639=VERTEX_POINT('',#9767);
#2640=VERTEX_POINT('',#9804);
#2641=VERTEX_POINT('',#9805);
#2642=VERTEX_POINT('',#9843);
#2643=VERTEX_POINT('',#9844);
#2644=VERTEX_POINT('',#9855);
#2645=VERTEX_POINT('',#9886);
#2646=VERTEX_POINT('',#9888);
#2647=VERTEX_POINT('',#9899);
#2648=VERTEX_POINT('',#9929);
#2649=VERTEX_POINT('',#9932);
#2650=VERTEX_POINT('',#9935);
#2651=VERTEX_POINT('',#9936);
#2652=VERTEX_POINT('',#9955);
#2653=VERTEX_POINT('',#9976);
#2654=VERTEX_POINT('',#9977);
#2655=VERTEX_POINT('',#9996);
#2656=VERTEX_POINT('',#10023);
#2657=VERTEX_POINT('',#10025);
#2658=VERTEX_POINT('',#10026);
#2659=VERTEX_POINT('',#10028);
#2660=VERTEX_POINT('',#10030);
#2661=VERTEX_POINT('',#10032);
#2662=VERTEX_POINT('',#10034);
#2663=VERTEX_POINT('',#10036);
#2664=VERTEX_POINT('',#10038);
#2665=VERTEX_POINT('',#10040);
#2666=VERTEX_POINT('',#10042);
#2667=VERTEX_POINT('',#10044);
#2668=VERTEX_POINT('',#10046);
#2669=VERTEX_POINT('',#10048);
#2670=VERTEX_POINT('',#10050);
#2671=VERTEX_POINT('',#10052);
#2672=VERTEX_POINT('',#10054);
#2673=VERTEX_POINT('',#10056);
#2674=VERTEX_POINT('',#10058);
#2675=VERTEX_POINT('',#10060);
#2676=VERTEX_POINT('',#10062);
#2677=VERTEX_POINT('',#10064);
#2678=VERTEX_POINT('',#10066);
#2679=VERTEX_POINT('',#10068);
#2680=VERTEX_POINT('',#10070);
#2681=VERTEX_POINT('',#10072);
#2682=VERTEX_POINT('',#10074);
#2683=VERTEX_POINT('',#10076);
#2684=VERTEX_POINT('',#10078);
#2685=VERTEX_POINT('',#10080);
#2686=VERTEX_POINT('',#10082);
#2687=VERTEX_POINT('',#10084);
#2688=VERTEX_POINT('',#10086);
#2689=VERTEX_POINT('',#10088);
#2690=VERTEX_POINT('',#10090);
#2691=VERTEX_POINT('',#10092);
#2692=VERTEX_POINT('',#10094);
#2693=VERTEX_POINT('',#10096);
#2694=VERTEX_POINT('',#10098);
#2695=VERTEX_POINT('',#10100);
#2696=VERTEX_POINT('',#10102);
#2697=VERTEX_POINT('',#10104);
#2698=VERTEX_POINT('',#10106);
#2699=VERTEX_POINT('',#10108);
#2700=VERTEX_POINT('',#10110);
#2701=VERTEX_POINT('',#10112);
#2702=VERTEX_POINT('',#10114);
#2703=VERTEX_POINT('',#10116);
#2704=VERTEX_POINT('',#10118);
#2705=VERTEX_POINT('',#10120);
#2706=VERTEX_POINT('',#10122);
#2707=VERTEX_POINT('',#10124);
#2708=VERTEX_POINT('',#10126);
#2709=VERTEX_POINT('',#10128);
#2710=VERTEX_POINT('',#10130);
#2711=VERTEX_POINT('',#10132);
#2712=VERTEX_POINT('',#10134);
#2713=VERTEX_POINT('',#10136);
#2714=VERTEX_POINT('',#10138);
#2715=VERTEX_POINT('',#10140);
#2716=VERTEX_POINT('',#10142);
#2717=VERTEX_POINT('',#10144);
#2718=VERTEX_POINT('',#10146);
#2719=VERTEX_POINT('',#10148);
#2720=VERTEX_POINT('',#10150);
#2721=VERTEX_POINT('',#10152);
#2722=VERTEX_POINT('',#10154);
#2723=VERTEX_POINT('',#10156);
#2724=VERTEX_POINT('',#10158);
#2725=VERTEX_POINT('',#10160);
#2726=VERTEX_POINT('',#10162);
#2727=VERTEX_POINT('',#10164);
#2728=VERTEX_POINT('',#10166);
#2729=VERTEX_POINT('',#10168);
#2730=VERTEX_POINT('',#10170);
#2731=VERTEX_POINT('',#10172);
#2732=VERTEX_POINT('',#10174);
#2733=VERTEX_POINT('',#10176);
#2734=VERTEX_POINT('',#10178);
#2735=VERTEX_POINT('',#10180);
#2736=VERTEX_POINT('',#10182);
#2737=VERTEX_POINT('',#10186);
#2738=VERTEX_POINT('',#10191);
#2739=VERTEX_POINT('',#10193);
#2740=VERTEX_POINT('',#10194);
#2741=VERTEX_POINT('',#10196);
#2742=VERTEX_POINT('',#10198);
#2743=VERTEX_POINT('',#10200);
#2744=VERTEX_POINT('',#10202);
#2745=VERTEX_POINT('',#10204);
#2746=VERTEX_POINT('',#10206);
#2747=VERTEX_POINT('',#10208);
#2748=VERTEX_POINT('',#10210);
#2749=VERTEX_POINT('',#10212);
#2750=VERTEX_POINT('',#10214);
#2751=VERTEX_POINT('',#10216);
#2752=VERTEX_POINT('',#10218);
#2753=VERTEX_POINT('',#10220);
#2754=VERTEX_POINT('',#10222);
#2755=VERTEX_POINT('',#10224);
#2756=VERTEX_POINT('',#10226);
#2757=VERTEX_POINT('',#10228);
#2758=VERTEX_POINT('',#10230);
#2759=VERTEX_POINT('',#10232);
#2760=VERTEX_POINT('',#10234);
#2761=VERTEX_POINT('',#10236);
#2762=VERTEX_POINT('',#10238);
#2763=VERTEX_POINT('',#10240);
#2764=VERTEX_POINT('',#10242);
#2765=VERTEX_POINT('',#10244);
#2766=VERTEX_POINT('',#10246);
#2767=VERTEX_POINT('',#10248);
#2768=VERTEX_POINT('',#10250);
#2769=VERTEX_POINT('',#10252);
#2770=VERTEX_POINT('',#10254);
#2771=VERTEX_POINT('',#10256);
#2772=VERTEX_POINT('',#10258);
#2773=VERTEX_POINT('',#10260);
#2774=VERTEX_POINT('',#10262);
#2775=VERTEX_POINT('',#10264);
#2776=VERTEX_POINT('',#10266);
#2777=VERTEX_POINT('',#10268);
#2778=VERTEX_POINT('',#10270);
#2779=VERTEX_POINT('',#10272);
#2780=VERTEX_POINT('',#10274);
#2781=VERTEX_POINT('',#10276);
#2782=VERTEX_POINT('',#10278);
#2783=VERTEX_POINT('',#10280);
#2784=VERTEX_POINT('',#10282);
#2785=VERTEX_POINT('',#10284);
#2786=VERTEX_POINT('',#10286);
#2787=VERTEX_POINT('',#10288);
#2788=VERTEX_POINT('',#10290);
#2789=VERTEX_POINT('',#10292);
#2790=VERTEX_POINT('',#10294);
#2791=VERTEX_POINT('',#10296);
#2792=VERTEX_POINT('',#10298);
#2793=VERTEX_POINT('',#10300);
#2794=VERTEX_POINT('',#10302);
#2795=VERTEX_POINT('',#10304);
#2796=VERTEX_POINT('',#10306);
#2797=VERTEX_POINT('',#10308);
#2798=VERTEX_POINT('',#10310);
#2799=VERTEX_POINT('',#10312);
#2800=VERTEX_POINT('',#10314);
#2801=VERTEX_POINT('',#10316);
#2802=VERTEX_POINT('',#10318);
#2803=VERTEX_POINT('',#10320);
#2804=VERTEX_POINT('',#10322);
#2805=VERTEX_POINT('',#10324);
#2806=VERTEX_POINT('',#10326);
#2807=VERTEX_POINT('',#10328);
#2808=VERTEX_POINT('',#10330);
#2809=VERTEX_POINT('',#10332);
#2810=VERTEX_POINT('',#10334);
#2811=VERTEX_POINT('',#10336);
#2812=VERTEX_POINT('',#10338);
#2813=VERTEX_POINT('',#10340);
#2814=VERTEX_POINT('',#10342);
#2815=VERTEX_POINT('',#10344);
#2816=VERTEX_POINT('',#10346);
#2817=VERTEX_POINT('',#10348);
#2818=VERTEX_POINT('',#10350);
#3239=EDGE_CURVE('',#2626,#2627,#1505,.T.);
#3240=EDGE_CURVE('',#2626,#2628,#1506,.T.);
#3241=EDGE_CURVE('',#2629,#2628,#1507,.T.);
#3242=EDGE_CURVE('',#2627,#2629,#1508,.T.);
#3243=EDGE_CURVE('',#2630,#2626,#1509,.T.);
#3244=EDGE_CURVE('',#2630,#2631,#1510,.T.);
#3245=EDGE_CURVE('',#2628,#2631,#1511,.T.);
#3246=EDGE_CURVE('',#2632,#2632,#2203,.T.);
#3247=EDGE_CURVE('',#2633,#2630,#1512,.T.);
#3248=EDGE_CURVE('',#2634,#2633,#1513,.T.);
#3249=EDGE_CURVE('',#2631,#2634,#1514,.T.);
#3250=EDGE_CURVE('',#2635,#2635,#2204,.T.);
#3251=EDGE_CURVE('',#2634,#2629,#2205,.T.);
#3252=EDGE_CURVE('',#2627,#2633,#2206,.T.);
#3253=EDGE_CURVE('',#2636,#2637,#220,.T.);
#3254=EDGE_CURVE('',#2637,#2636,#221,.T.);
#3255=EDGE_CURVE('',#2638,#2639,#222,.T.);
#3256=EDGE_CURVE('',#2639,#2638,#223,.T.);
#3257=EDGE_CURVE('',#2640,#2641,#224,.T.);
#3258=EDGE_CURVE('',#2641,#2640,#225,.T.);
#3259=EDGE_CURVE('',#2642,#2643,#226,.T.);
#3260=EDGE_CURVE('',#2644,#2642,#227,.T.);
#3261=EDGE_CURVE('',#2643,#2644,#228,.T.);
#3262=EDGE_CURVE('',#2643,#2639,#1515,.T.);
#3263=EDGE_CURVE('',#2641,#2645,#1516,.T.);
#3264=EDGE_CURVE('',#2646,#2645,#229,.T.);
#3265=EDGE_CURVE('',#2647,#2646,#230,.T.);
#3266=EDGE_CURVE('',#2645,#2647,#231,.T.);
#3267=EDGE_CURVE('',#2648,#2648,#2207,.T.);
#3268=EDGE_CURVE('',#2648,#2644,#1517,.T.);
#3269=EDGE_CURVE('',#2642,#2649,#1518,.T.);
#3270=EDGE_CURVE('',#2649,#2649,#2208,.T.);
#3271=EDGE_CURVE('',#2650,#2651,#232,.T.);
#3272=EDGE_CURVE('',#2651,#2652,#233,.T.);
#3273=EDGE_CURVE('',#2652,#2650,#234,.T.);
#3274=EDGE_CURVE('',#2653,#2654,#235,.T.);
#3275=EDGE_CURVE('',#2654,#2655,#236,.T.);
#3276=EDGE_CURVE('',#2655,#2653,#237,.T.);
#3277=EDGE_CURVE('',#2652,#2632,#1519,.T.);
#3278=EDGE_CURVE('',#2637,#2655,#1520,.T.);
#3279=EDGE_CURVE('',#2656,#2656,#2209,.T.);
#3280=EDGE_CURVE('',#2657,#2658,#2210,.T.);
#3281=EDGE_CURVE('',#2659,#2658,#2211,.T.);
#3282=EDGE_CURVE('',#2659,#2660,#2212,.T.);
#3283=EDGE_CURVE('',#2661,#2660,#2213,.T.);
#3284=EDGE_CURVE('',#2661,#2662,#2214,.T.);
#3285=EDGE_CURVE('',#2663,#2662,#2215,.T.);
#3286=EDGE_CURVE('',#2663,#2664,#2216,.T.);
#3287=EDGE_CURVE('',#2665,#2664,#2217,.T.);
#3288=EDGE_CURVE('',#2665,#2666,#2218,.T.);
#3289=EDGE_CURVE('',#2667,#2666,#2219,.T.);
#3290=EDGE_CURVE('',#2667,#2668,#2220,.T.);
#3291=EDGE_CURVE('',#2669,#2668,#2221,.T.);
#3292=EDGE_CURVE('',#2669,#2670,#2222,.T.);
#3293=EDGE_CURVE('',#2671,#2670,#2223,.T.);
#3294=EDGE_CURVE('',#2671,#2672,#2224,.T.);
#3295=EDGE_CURVE('',#2673,#2672,#2225,.T.);
#3296=EDGE_CURVE('',#2673,#2674,#2226,.T.);
#3297=EDGE_CURVE('',#2675,#2674,#2227,.T.);
#3298=EDGE_CURVE('',#2675,#2676,#2228,.T.);
#3299=EDGE_CURVE('',#2677,#2676,#2229,.T.);
#3300=EDGE_CURVE('',#2677,#2678,#2230,.T.);
#3301=EDGE_CURVE('',#2679,#2678,#2231,.T.);
#3302=EDGE_CURVE('',#2679,#2680,#2232,.T.);
#3303=EDGE_CURVE('',#2681,#2680,#2233,.T.);
#3304=EDGE_CURVE('',#2681,#2682,#2234,.T.);
#3305=EDGE_CURVE('',#2683,#2682,#2235,.T.);
#3306=EDGE_CURVE('',#2683,#2684,#2236,.T.);
#3307=EDGE_CURVE('',#2685,#2684,#2237,.T.);
#3308=EDGE_CURVE('',#2685,#2686,#2238,.T.);
#3309=EDGE_CURVE('',#2687,#2686,#2239,.T.);
#3310=EDGE_CURVE('',#2687,#2688,#2240,.T.);
#3311=EDGE_CURVE('',#2689,#2688,#2241,.T.);
#3312=EDGE_CURVE('',#2689,#2690,#2242,.T.);
#3313=EDGE_CURVE('',#2691,#2690,#2243,.T.);
#3314=EDGE_CURVE('',#2691,#2692,#2244,.T.);
#3315=EDGE_CURVE('',#2693,#2692,#2245,.T.);
#3316=EDGE_CURVE('',#2693,#2694,#2246,.T.);
#3317=EDGE_CURVE('',#2695,#2694,#2247,.T.);
#3318=EDGE_CURVE('',#2695,#2696,#2248,.T.);
#3319=EDGE_CURVE('',#2697,#2696,#2249,.T.);
#3320=EDGE_CURVE('',#2697,#2698,#2250,.T.);
#3321=EDGE_CURVE('',#2699,#2698,#2251,.T.);
#3322=EDGE_CURVE('',#2699,#2700,#2252,.T.);
#3323=EDGE_CURVE('',#2701,#2700,#2253,.T.);
#3324=EDGE_CURVE('',#2701,#2702,#2254,.T.);
#3325=EDGE_CURVE('',#2703,#2702,#2255,.T.);
#3326=EDGE_CURVE('',#2703,#2704,#2256,.T.);
#3327=EDGE_CURVE('',#2705,#2704,#2257,.T.);
#3328=EDGE_CURVE('',#2705,#2706,#2258,.T.);
#3329=EDGE_CURVE('',#2707,#2706,#2259,.T.);
#3330=EDGE_CURVE('',#2707,#2708,#2260,.T.);
#3331=EDGE_CURVE('',#2709,#2708,#2261,.T.);
#3332=EDGE_CURVE('',#2709,#2710,#2262,.T.);
#3333=EDGE_CURVE('',#2711,#2710,#2263,.T.);
#3334=EDGE_CURVE('',#2711,#2712,#2264,.T.);
#3335=EDGE_CURVE('',#2713,#2712,#2265,.T.);
#3336=EDGE_CURVE('',#2713,#2714,#2266,.T.);
#3337=EDGE_CURVE('',#2715,#2714,#2267,.T.);
#3338=EDGE_CURVE('',#2715,#2716,#2268,.T.);
#3339=EDGE_CURVE('',#2717,#2716,#2269,.T.);
#3340=EDGE_CURVE('',#2717,#2718,#2270,.T.);
#3341=EDGE_CURVE('',#2719,#2718,#2271,.T.);
#3342=EDGE_CURVE('',#2719,#2720,#2272,.T.);
#3343=EDGE_CURVE('',#2721,#2720,#2273,.T.);
#3344=EDGE_CURVE('',#2721,#2722,#2274,.T.);
#3345=EDGE_CURVE('',#2723,#2722,#2275,.T.);
#3346=EDGE_CURVE('',#2723,#2724,#2276,.T.);
#3347=EDGE_CURVE('',#2725,#2724,#2277,.T.);
#3348=EDGE_CURVE('',#2725,#2726,#2278,.T.);
#3349=EDGE_CURVE('',#2727,#2726,#2279,.T.);
#3350=EDGE_CURVE('',#2727,#2728,#2280,.T.);
#3351=EDGE_CURVE('',#2729,#2728,#2281,.T.);
#3352=EDGE_CURVE('',#2729,#2730,#2282,.T.);
#3353=EDGE_CURVE('',#2731,#2730,#2283,.T.);
#3354=EDGE_CURVE('',#2731,#2732,#2284,.T.);
#3355=EDGE_CURVE('',#2733,#2732,#2285,.T.);
#3356=EDGE_CURVE('',#2733,#2734,#2286,.T.);
#3357=EDGE_CURVE('',#2735,#2734,#2287,.T.);
#3358=EDGE_CURVE('',#2735,#2736,#2288,.T.);
#3359=EDGE_CURVE('',#2657,#2736,#2289,.T.);
#3360=EDGE_CURVE('',#2737,#2737,#2290,.T.);
#3361=EDGE_CURVE('',#2737,#2656,#1521,.T.);
#3362=EDGE_CURVE('',#2738,#2738,#2291,.T.);
#3363=EDGE_CURVE('',#2739,#2740,#2292,.T.);
#3364=EDGE_CURVE('',#2740,#2741,#2293,.T.);
#3365=EDGE_CURVE('',#2741,#2742,#2294,.T.);
#3366=EDGE_CURVE('',#2742,#2743,#2295,.T.);
#3367=EDGE_CURVE('',#2743,#2744,#2296,.T.);
#3368=EDGE_CURVE('',#2744,#2745,#2297,.T.);
#3369=EDGE_CURVE('',#2745,#2746,#2298,.T.);
#3370=EDGE_CURVE('',#2746,#2747,#2299,.T.);
#3371=EDGE_CURVE('',#2747,#2748,#2300,.T.);
#3372=EDGE_CURVE('',#2748,#2749,#2301,.T.);
#3373=EDGE_CURVE('',#2749,#2750,#2302,.T.);
#3374=EDGE_CURVE('',#2750,#2751,#2303,.T.);
#3375=EDGE_CURVE('',#2751,#2752,#2304,.T.);
#3376=EDGE_CURVE('',#2752,#2753,#2305,.T.);
#3377=EDGE_CURVE('',#2753,#2754,#2306,.T.);
#3378=EDGE_CURVE('',#2754,#2755,#2307,.T.);
#3379=EDGE_CURVE('',#2755,#2756,#2308,.T.);
#3380=EDGE_CURVE('',#2756,#2757,#2309,.T.);
#3381=EDGE_CURVE('',#2757,#2758,#2310,.T.);
#3382=EDGE_CURVE('',#2758,#2759,#2311,.T.);
#3383=EDGE_CURVE('',#2759,#2760,#2312,.T.);
#3384=EDGE_CURVE('',#2760,#2761,#2313,.T.);
#3385=EDGE_CURVE('',#2761,#2762,#2314,.T.);
#3386=EDGE_CURVE('',#2762,#2763,#2315,.T.);
#3387=EDGE_CURVE('',#2763,#2764,#2316,.T.);
#3388=EDGE_CURVE('',#2764,#2765,#2317,.T.);
#3389=EDGE_CURVE('',#2765,#2766,#2318,.T.);
#3390=EDGE_CURVE('',#2766,#2767,#2319,.T.);
#3391=EDGE_CURVE('',#2767,#2768,#2320,.T.);
#3392=EDGE_CURVE('',#2768,#2769,#2321,.T.);
#3393=EDGE_CURVE('',#2769,#2770,#2322,.T.);
#3394=EDGE_CURVE('',#2770,#2771,#2323,.T.);
#3395=EDGE_CURVE('',#2771,#2772,#2324,.T.);
#3396=EDGE_CURVE('',#2772,#2773,#2325,.T.);
#3397=EDGE_CURVE('',#2773,#2774,#2326,.T.);
#3398=EDGE_CURVE('',#2774,#2775,#2327,.T.);
#3399=EDGE_CURVE('',#2775,#2776,#2328,.T.);
#3400=EDGE_CURVE('',#2776,#2777,#2329,.T.);
#3401=EDGE_CURVE('',#2777,#2778,#2330,.T.);
#3402=EDGE_CURVE('',#2778,#2779,#2331,.T.);
#3403=EDGE_CURVE('',#2779,#2780,#2332,.T.);
#3404=EDGE_CURVE('',#2780,#2781,#2333,.T.);
#3405=EDGE_CURVE('',#2781,#2782,#2334,.T.);
#3406=EDGE_CURVE('',#2782,#2783,#2335,.T.);
#3407=EDGE_CURVE('',#2783,#2784,#2336,.T.);
#3408=EDGE_CURVE('',#2784,#2785,#2337,.T.);
#3409=EDGE_CURVE('',#2785,#2786,#2338,.T.);
#3410=EDGE_CURVE('',#2786,#2787,#2339,.T.);
#3411=EDGE_CURVE('',#2787,#2788,#2340,.T.);
#3412=EDGE_CURVE('',#2788,#2789,#2341,.T.);
#3413=EDGE_CURVE('',#2789,#2790,#2342,.T.);
#3414=EDGE_CURVE('',#2790,#2791,#2343,.T.);
#3415=EDGE_CURVE('',#2791,#2792,#2344,.T.);
#3416=EDGE_CURVE('',#2792,#2793,#2345,.T.);
#3417=EDGE_CURVE('',#2793,#2794,#2346,.T.);
#3418=EDGE_CURVE('',#2794,#2795,#2347,.T.);
#3419=EDGE_CURVE('',#2795,#2796,#2348,.T.);
#3420=EDGE_CURVE('',#2796,#2797,#2349,.T.);
#3421=EDGE_CURVE('',#2797,#2798,#2350,.T.);
#3422=EDGE_CURVE('',#2798,#2799,#2351,.T.);
#3423=EDGE_CURVE('',#2799,#2800,#2352,.T.);
#3424=EDGE_CURVE('',#2800,#2801,#2353,.T.);
#3425=EDGE_CURVE('',#2801,#2802,#2354,.T.);
#3426=EDGE_CURVE('',#2802,#2803,#2355,.T.);
#3427=EDGE_CURVE('',#2803,#2804,#2356,.T.);
#3428=EDGE_CURVE('',#2804,#2805,#2357,.T.);
#3429=EDGE_CURVE('',#2805,#2806,#2358,.T.);
#3430=EDGE_CURVE('',#2806,#2807,#2359,.T.);
#3431=EDGE_CURVE('',#2807,#2808,#2360,.T.);
#3432=EDGE_CURVE('',#2808,#2809,#2361,.T.);
#3433=EDGE_CURVE('',#2809,#2810,#2362,.T.);
#3434=EDGE_CURVE('',#2810,#2811,#2363,.T.);
#3435=EDGE_CURVE('',#2811,#2812,#2364,.T.);
#3436=EDGE_CURVE('',#2812,#2813,#2365,.T.);
#3437=EDGE_CURVE('',#2813,#2814,#2366,.T.);
#3438=EDGE_CURVE('',#2814,#2815,#2367,.T.);
#3439=EDGE_CURVE('',#2815,#2816,#2368,.T.);
#3440=EDGE_CURVE('',#2816,#2817,#2369,.T.);
#3441=EDGE_CURVE('',#2817,#2818,#2370,.T.);
#3442=EDGE_CURVE('',#2818,#2739,#2371,.T.);
#3443=EDGE_CURVE('',#2635,#2738,#1522,.T.);
#3444=EDGE_CURVE('',#2740,#2657,#1523,.T.);
#3445=EDGE_CURVE('',#2658,#2739,#1524,.T.);
#3446=EDGE_CURVE('',#2818,#2659,#1525,.T.);
#3447=EDGE_CURVE('',#2660,#2817,#1526,.T.);
#3448=EDGE_CURVE('',#2816,#2661,#1527,.T.);
#3449=EDGE_CURVE('',#2662,#2815,#1528,.T.);
#3450=EDGE_CURVE('',#2814,#2663,#1529,.T.);
#3451=EDGE_CURVE('',#2664,#2813,#1530,.T.);
#3452=EDGE_CURVE('',#2812,#2665,#1531,.T.);
#3453=EDGE_CURVE('',#2666,#2811,#1532,.T.);
#3454=EDGE_CURVE('',#2810,#2667,#1533,.T.);
#3455=EDGE_CURVE('',#2668,#2809,#1534,.T.);
#3456=EDGE_CURVE('',#2808,#2669,#1535,.T.);
#3457=EDGE_CURVE('',#2670,#2807,#1536,.T.);
#3458=EDGE_CURVE('',#2806,#2671,#1537,.T.);
#3459=EDGE_CURVE('',#2672,#2805,#1538,.T.);
#3460=EDGE_CURVE('',#2804,#2673,#1539,.T.);
#3461=EDGE_CURVE('',#2674,#2803,#1540,.T.);
#3462=EDGE_CURVE('',#2802,#2675,#1541,.T.);
#3463=EDGE_CURVE('',#2676,#2801,#1542,.T.);
#3464=EDGE_CURVE('',#2800,#2677,#1543,.T.);
#3465=EDGE_CURVE('',#2678,#2799,#1544,.T.);
#3466=EDGE_CURVE('',#2798,#2679,#1545,.T.);
#3467=EDGE_CURVE('',#2680,#2797,#1546,.T.);
#3468=EDGE_CURVE('',#2796,#2681,#1547,.T.);
#3469=EDGE_CURVE('',#2682,#2795,#1548,.T.);
#3470=EDGE_CURVE('',#2794,#2683,#1549,.T.);
#3471=EDGE_CURVE('',#2684,#2793,#1550,.T.);
#3472=EDGE_CURVE('',#2792,#2685,#1551,.T.);
#3473=EDGE_CURVE('',#2686,#2791,#1552,.T.);
#3474=EDGE_CURVE('',#2790,#2687,#1553,.T.);
#3475=EDGE_CURVE('',#2688,#2789,#1554,.T.);
#3476=EDGE_CURVE('',#2788,#2689,#1555,.T.);
#3477=EDGE_CURVE('',#2690,#2787,#1556,.T.);
#3478=EDGE_CURVE('',#2786,#2691,#1557,.T.);
#3479=EDGE_CURVE('',#2692,#2785,#1558,.T.);
#3480=EDGE_CURVE('',#2784,#2693,#1559,.T.);
#3481=EDGE_CURVE('',#2694,#2783,#1560,.T.);
#3482=EDGE_CURVE('',#2782,#2695,#1561,.T.);
#3483=EDGE_CURVE('',#2696,#2781,#1562,.T.);
#3484=EDGE_CURVE('',#2780,#2697,#1563,.T.);
#3485=EDGE_CURVE('',#2698,#2779,#1564,.T.);
#3486=EDGE_CURVE('',#2778,#2699,#1565,.T.);
#3487=EDGE_CURVE('',#2700,#2777,#1566,.T.);
#3488=EDGE_CURVE('',#2776,#2701,#1567,.T.);
#3489=EDGE_CURVE('',#2702,#2775,#1568,.T.);
#3490=EDGE_CURVE('',#2774,#2703,#1569,.T.);
#3491=EDGE_CURVE('',#2704,#2773,#1570,.T.);
#3492=EDGE_CURVE('',#2772,#2705,#1571,.T.);
#3493=EDGE_CURVE('',#2706,#2771,#1572,.T.);
#3494=EDGE_CURVE('',#2770,#2707,#1573,.T.);
#3495=EDGE_CURVE('',#2708,#2769,#1574,.T.);
#3496=EDGE_CURVE('',#2768,#2709,#1575,.T.);
#3497=EDGE_CURVE('',#2710,#2767,#1576,.T.);
#3498=EDGE_CURVE('',#2766,#2711,#1577,.T.);
#3499=EDGE_CURVE('',#2712,#2765,#1578,.T.);
#3500=EDGE_CURVE('',#2764,#2713,#1579,.T.);
#3501=EDGE_CURVE('',#2714,#2763,#1580,.T.);
#3502=EDGE_CURVE('',#2762,#2715,#1581,.T.);
#3503=EDGE_CURVE('',#2716,#2761,#1582,.T.);
#3504=EDGE_CURVE('',#2760,#2717,#1583,.T.);
#3505=EDGE_CURVE('',#2718,#2759,#1584,.T.);
#3506=EDGE_CURVE('',#2758,#2719,#1585,.T.);
#3507=EDGE_CURVE('',#2720,#2757,#1586,.T.);
#3508=EDGE_CURVE('',#2756,#2721,#1587,.T.);
#3509=EDGE_CURVE('',#2722,#2755,#1588,.T.);
#3510=EDGE_CURVE('',#2754,#2723,#1589,.T.);
#3511=EDGE_CURVE('',#2724,#2753,#1590,.T.);
#3512=EDGE_CURVE('',#2752,#2725,#1591,.T.);
#3513=EDGE_CURVE('',#2726,#2751,#1592,.T.);
#3514=EDGE_CURVE('',#2750,#2727,#1593,.T.);
#3515=EDGE_CURVE('',#2728,#2749,#1594,.T.);
#3516=EDGE_CURVE('',#2748,#2729,#1595,.T.);
#3517=EDGE_CURVE('',#2730,#2747,#1596,.T.);
#3518=EDGE_CURVE('',#2746,#2731,#1597,.T.);
#3519=EDGE_CURVE('',#2732,#2745,#1598,.T.);
#3520=EDGE_CURVE('',#2744,#2733,#1599,.T.);
#3521=EDGE_CURVE('',#2734,#2743,#1600,.T.);
#3522=EDGE_CURVE('',#2736,#2741,#1601,.T.);
#3523=EDGE_CURVE('',#2742,#2735,#1602,.T.);
#4333=ORIENTED_EDGE('',*,*,#3239,.F.);
#4334=ORIENTED_EDGE('',*,*,#3240,.T.);
#4335=ORIENTED_EDGE('',*,*,#3241,.F.);
#4336=ORIENTED_EDGE('',*,*,#3242,.F.);
#4337=ORIENTED_EDGE('',*,*,#3243,.F.);
#4338=ORIENTED_EDGE('',*,*,#3244,.T.);
#4339=ORIENTED_EDGE('',*,*,#3245,.F.);
#4340=ORIENTED_EDGE('',*,*,#3240,.F.);
#4341=ORIENTED_EDGE('',*,*,#3246,.F.);
#4342=ORIENTED_EDGE('',*,*,#3247,.F.);
#4343=ORIENTED_EDGE('',*,*,#3248,.F.);
#4344=ORIENTED_EDGE('',*,*,#3249,.F.);
#4345=ORIENTED_EDGE('',*,*,#3244,.F.);
#4346=ORIENTED_EDGE('',*,*,#3250,.T.);
#4347=ORIENTED_EDGE('',*,*,#3241,.T.);
#4348=ORIENTED_EDGE('',*,*,#3245,.T.);
#4349=ORIENTED_EDGE('',*,*,#3249,.T.);
#4350=ORIENTED_EDGE('',*,*,#3251,.T.);
#4351=ORIENTED_EDGE('',*,*,#3242,.T.);
#4352=ORIENTED_EDGE('',*,*,#3251,.F.);
#4353=ORIENTED_EDGE('',*,*,#3248,.T.);
#4354=ORIENTED_EDGE('',*,*,#3252,.F.);
#4355=ORIENTED_EDGE('',*,*,#3253,.T.);
#4356=ORIENTED_EDGE('',*,*,#3254,.T.);
#4357=ORIENTED_EDGE('',*,*,#3255,.T.);
#4358=ORIENTED_EDGE('',*,*,#3256,.T.);
#4359=ORIENTED_EDGE('',*,*,#3257,.T.);
#4360=ORIENTED_EDGE('',*,*,#3258,.T.);
#4361=ORIENTED_EDGE('',*,*,#3259,.F.);
#4362=ORIENTED_EDGE('',*,*,#3260,.F.);
#4363=ORIENTED_EDGE('',*,*,#3261,.F.);
#4364=ORIENTED_EDGE('',*,*,#3262,.T.);
#4365=ORIENTED_EDGE('',*,*,#3255,.F.);
#4366=ORIENTED_EDGE('',*,*,#3256,.F.);
#4367=ORIENTED_EDGE('',*,*,#3262,.F.);
#4368=ORIENTED_EDGE('',*,*,#3257,.F.);
#4369=ORIENTED_EDGE('',*,*,#3258,.F.);
#4370=ORIENTED_EDGE('',*,*,#3263,.T.);
#4371=ORIENTED_EDGE('',*,*,#3264,.F.);
#4372=ORIENTED_EDGE('',*,*,#3265,.F.);
#4373=ORIENTED_EDGE('',*,*,#3266,.F.);
#4374=ORIENTED_EDGE('',*,*,#3263,.F.);
#4375=ORIENTED_EDGE('',*,*,#3267,.F.);
#4376=ORIENTED_EDGE('',*,*,#3268,.T.);
#4377=ORIENTED_EDGE('',*,*,#3260,.T.);
#4378=ORIENTED_EDGE('',*,*,#3269,.T.);
#4379=ORIENTED_EDGE('',*,*,#3270,.F.);
#4380=ORIENTED_EDGE('',*,*,#3269,.F.);
#4381=ORIENTED_EDGE('',*,*,#3259,.T.);
#4382=ORIENTED_EDGE('',*,*,#3261,.T.);
#4383=ORIENTED_EDGE('',*,*,#3268,.F.);
#4384=ORIENTED_EDGE('',*,*,#3265,.T.);
#4385=ORIENTED_EDGE('',*,*,#3264,.T.);
#4386=ORIENTED_EDGE('',*,*,#3266,.T.);
#4387=ORIENTED_EDGE('',*,*,#3271,.T.);
#4388=ORIENTED_EDGE('',*,*,#3272,.T.);
#4389=ORIENTED_EDGE('',*,*,#3273,.T.);
#4390=ORIENTED_EDGE('',*,*,#3274,.T.);
#4391=ORIENTED_EDGE('',*,*,#3275,.T.);
#4392=ORIENTED_EDGE('',*,*,#3276,.T.);
#4393=ORIENTED_EDGE('',*,*,#3272,.F.);
#4394=ORIENTED_EDGE('',*,*,#3271,.F.);
#4395=ORIENTED_EDGE('',*,*,#3273,.F.);
#4396=ORIENTED_EDGE('',*,*,#3277,.T.);
#4397=ORIENTED_EDGE('',*,*,#3246,.T.);
#4398=ORIENTED_EDGE('',*,*,#3277,.F.);
#4399=ORIENTED_EDGE('',*,*,#3253,.F.);
#4400=ORIENTED_EDGE('',*,*,#3254,.F.);
#4401=ORIENTED_EDGE('',*,*,#3278,.T.);
#4402=ORIENTED_EDGE('',*,*,#3275,.F.);
#4403=ORIENTED_EDGE('',*,*,#3274,.F.);
#4404=ORIENTED_EDGE('',*,*,#3276,.F.);
#4405=ORIENTED_EDGE('',*,*,#3278,.F.);
#4406=ORIENTED_EDGE('',*,*,#3267,.T.);
#4407=ORIENTED_EDGE('',*,*,#3239,.T.);
#4408=ORIENTED_EDGE('',*,*,#3252,.T.);
#4409=ORIENTED_EDGE('',*,*,#3247,.T.);
#4410=ORIENTED_EDGE('',*,*,#3243,.T.);
#4411=ORIENTED_EDGE('',*,*,#3279,.T.);
#4412=ORIENTED_EDGE('',*,*,#3280,.T.);
#4413=ORIENTED_EDGE('',*,*,#3281,.F.);
#4414=ORIENTED_EDGE('',*,*,#3282,.T.);
#4415=ORIENTED_EDGE('',*,*,#3283,.F.);
#4416=ORIENTED_EDGE('',*,*,#3284,.T.);
#4417=ORIENTED_EDGE('',*,*,#3285,.F.);
#4418=ORIENTED_EDGE('',*,*,#3286,.T.);
#4419=ORIENTED_EDGE('',*,*,#3287,.F.);
#4420=ORIENTED_EDGE('',*,*,#3288,.T.);
#4421=ORIENTED_EDGE('',*,*,#3289,.F.);
#4422=ORIENTED_EDGE('',*,*,#3290,.T.);
#4423=ORIENTED_EDGE('',*,*,#3291,.F.);
#4424=ORIENTED_EDGE('',*,*,#3292,.T.);
#4425=ORIENTED_EDGE('',*,*,#3293,.F.);
#4426=ORIENTED_EDGE('',*,*,#3294,.T.);
#4427=ORIENTED_EDGE('',*,*,#3295,.F.);
#4428=ORIENTED_EDGE('',*,*,#3296,.T.);
#4429=ORIENTED_EDGE('',*,*,#3297,.F.);
#4430=ORIENTED_EDGE('',*,*,#3298,.T.);
#4431=ORIENTED_EDGE('',*,*,#3299,.F.);
#4432=ORIENTED_EDGE('',*,*,#3300,.T.);
#4433=ORIENTED_EDGE('',*,*,#3301,.F.);
#4434=ORIENTED_EDGE('',*,*,#3302,.T.);
#4435=ORIENTED_EDGE('',*,*,#3303,.F.);
#4436=ORIENTED_EDGE('',*,*,#3304,.T.);
#4437=ORIENTED_EDGE('',*,*,#3305,.F.);
#4438=ORIENTED_EDGE('',*,*,#3306,.T.);
#4439=ORIENTED_EDGE('',*,*,#3307,.F.);
#4440=ORIENTED_EDGE('',*,*,#3308,.T.);
#4441=ORIENTED_EDGE('',*,*,#3309,.F.);
#4442=ORIENTED_EDGE('',*,*,#3310,.T.);
#4443=ORIENTED_EDGE('',*,*,#3311,.F.);
#4444=ORIENTED_EDGE('',*,*,#3312,.T.);
#4445=ORIENTED_EDGE('',*,*,#3313,.F.);
#4446=ORIENTED_EDGE('',*,*,#3314,.T.);
#4447=ORIENTED_EDGE('',*,*,#3315,.F.);
#4448=ORIENTED_EDGE('',*,*,#3316,.T.);
#4449=ORIENTED_EDGE('',*,*,#3317,.F.);
#4450=ORIENTED_EDGE('',*,*,#3318,.T.);
#4451=ORIENTED_EDGE('',*,*,#3319,.F.);
#4452=ORIENTED_EDGE('',*,*,#3320,.T.);
#4453=ORIENTED_EDGE('',*,*,#3321,.F.);
#4454=ORIENTED_EDGE('',*,*,#3322,.T.);
#4455=ORIENTED_EDGE('',*,*,#3323,.F.);
#4456=ORIENTED_EDGE('',*,*,#3324,.T.);
#4457=ORIENTED_EDGE('',*,*,#3325,.F.);
#4458=ORIENTED_EDGE('',*,*,#3326,.T.);
#4459=ORIENTED_EDGE('',*,*,#3327,.F.);
#4460=ORIENTED_EDGE('',*,*,#3328,.T.);
#4461=ORIENTED_EDGE('',*,*,#3329,.F.);
#4462=ORIENTED_EDGE('',*,*,#3330,.T.);
#4463=ORIENTED_EDGE('',*,*,#3331,.F.);
#4464=ORIENTED_EDGE('',*,*,#3332,.T.);
#4465=ORIENTED_EDGE('',*,*,#3333,.F.);
#4466=ORIENTED_EDGE('',*,*,#3334,.T.);
#4467=ORIENTED_EDGE('',*,*,#3335,.F.);
#4468=ORIENTED_EDGE('',*,*,#3336,.T.);
#4469=ORIENTED_EDGE('',*,*,#3337,.F.);
#4470=ORIENTED_EDGE('',*,*,#3338,.T.);
#4471=ORIENTED_EDGE('',*,*,#3339,.F.);
#4472=ORIENTED_EDGE('',*,*,#3340,.T.);
#4473=ORIENTED_EDGE('',*,*,#3341,.F.);
#4474=ORIENTED_EDGE('',*,*,#3342,.T.);
#4475=ORIENTED_EDGE('',*,*,#3343,.F.);
#4476=ORIENTED_EDGE('',*,*,#3344,.T.);
#4477=ORIENTED_EDGE('',*,*,#3345,.F.);
#4478=ORIENTED_EDGE('',*,*,#3346,.T.);
#4479=ORIENTED_EDGE('',*,*,#3347,.F.);
#4480=ORIENTED_EDGE('',*,*,#3348,.T.);
#4481=ORIENTED_EDGE('',*,*,#3349,.F.);
#4482=ORIENTED_EDGE('',*,*,#3350,.T.);
#4483=ORIENTED_EDGE('',*,*,#3351,.F.);
#4484=ORIENTED_EDGE('',*,*,#3352,.T.);
#4485=ORIENTED_EDGE('',*,*,#3353,.F.);
#4486=ORIENTED_EDGE('',*,*,#3354,.T.);
#4487=ORIENTED_EDGE('',*,*,#3355,.F.);
#4488=ORIENTED_EDGE('',*,*,#3356,.T.);
#4489=ORIENTED_EDGE('',*,*,#3357,.F.);
#4490=ORIENTED_EDGE('',*,*,#3358,.T.);
#4491=ORIENTED_EDGE('',*,*,#3359,.F.);
#4492=ORIENTED_EDGE('',*,*,#3360,.F.);
#4493=ORIENTED_EDGE('',*,*,#3361,.T.);
#4494=ORIENTED_EDGE('',*,*,#3279,.F.);
#4495=ORIENTED_EDGE('',*,*,#3361,.F.);
#4496=ORIENTED_EDGE('',*,*,#3360,.T.);
#4497=ORIENTED_EDGE('',*,*,#3270,.T.);
#4498=ORIENTED_EDGE('',*,*,#3362,.F.);
#4499=ORIENTED_EDGE('',*,*,#3363,.T.);
#4500=ORIENTED_EDGE('',*,*,#3364,.T.);
#4501=ORIENTED_EDGE('',*,*,#3365,.T.);
#4502=ORIENTED_EDGE('',*,*,#3366,.T.);
#4503=ORIENTED_EDGE('',*,*,#3367,.T.);
#4504=ORIENTED_EDGE('',*,*,#3368,.T.);
#4505=ORIENTED_EDGE('',*,*,#3369,.T.);
#4506=ORIENTED_EDGE('',*,*,#3370,.T.);
#4507=ORIENTED_EDGE('',*,*,#3371,.T.);
#4508=ORIENTED_EDGE('',*,*,#3372,.T.);
#4509=ORIENTED_EDGE('',*,*,#3373,.T.);
#4510=ORIENTED_EDGE('',*,*,#3374,.T.);
#4511=ORIENTED_EDGE('',*,*,#3375,.T.);
#4512=ORIENTED_EDGE('',*,*,#3376,.T.);
#4513=ORIENTED_EDGE('',*,*,#3377,.T.);
#4514=ORIENTED_EDGE('',*,*,#3378,.T.);
#4515=ORIENTED_EDGE('',*,*,#3379,.T.);
#4516=ORIENTED_EDGE('',*,*,#3380,.T.);
#4517=ORIENTED_EDGE('',*,*,#3381,.T.);
#4518=ORIENTED_EDGE('',*,*,#3382,.T.);
#4519=ORIENTED_EDGE('',*,*,#3383,.T.);
#4520=ORIENTED_EDGE('',*,*,#3384,.T.);
#4521=ORIENTED_EDGE('',*,*,#3385,.T.);
#4522=ORIENTED_EDGE('',*,*,#3386,.T.);
#4523=ORIENTED_EDGE('',*,*,#3387,.T.);
#4524=ORIENTED_EDGE('',*,*,#3388,.T.);
#4525=ORIENTED_EDGE('',*,*,#3389,.T.);
#4526=ORIENTED_EDGE('',*,*,#3390,.T.);
#4527=ORIENTED_EDGE('',*,*,#3391,.T.);
#4528=ORIENTED_EDGE('',*,*,#3392,.T.);
#4529=ORIENTED_EDGE('',*,*,#3393,.T.);
#4530=ORIENTED_EDGE('',*,*,#3394,.T.);
#4531=ORIENTED_EDGE('',*,*,#3395,.T.);
#4532=ORIENTED_EDGE('',*,*,#3396,.T.);
#4533=ORIENTED_EDGE('',*,*,#3397,.T.);
#4534=ORIENTED_EDGE('',*,*,#3398,.T.);
#4535=ORIENTED_EDGE('',*,*,#3399,.T.);
#4536=ORIENTED_EDGE('',*,*,#3400,.T.);
#4537=ORIENTED_EDGE('',*,*,#3401,.T.);
#4538=ORIENTED_EDGE('',*,*,#3402,.T.);
#4539=ORIENTED_EDGE('',*,*,#3403,.T.);
#4540=ORIENTED_EDGE('',*,*,#3404,.T.);
#4541=ORIENTED_EDGE('',*,*,#3405,.T.);
#4542=ORIENTED_EDGE('',*,*,#3406,.T.);
#4543=ORIENTED_EDGE('',*,*,#3407,.T.);
#4544=ORIENTED_EDGE('',*,*,#3408,.T.);
#4545=ORIENTED_EDGE('',*,*,#3409,.T.);
#4546=ORIENTED_EDGE('',*,*,#3410,.T.);
#4547=ORIENTED_EDGE('',*,*,#3411,.T.);
#4548=ORIENTED_EDGE('',*,*,#3412,.T.);
#4549=ORIENTED_EDGE('',*,*,#3413,.T.);
#4550=ORIENTED_EDGE('',*,*,#3414,.T.);
#4551=ORIENTED_EDGE('',*,*,#3415,.T.);
#4552=ORIENTED_EDGE('',*,*,#3416,.T.);
#4553=ORIENTED_EDGE('',*,*,#3417,.T.);
#4554=ORIENTED_EDGE('',*,*,#3418,.T.);
#4555=ORIENTED_EDGE('',*,*,#3419,.T.);
#4556=ORIENTED_EDGE('',*,*,#3420,.T.);
#4557=ORIENTED_EDGE('',*,*,#3421,.T.);
#4558=ORIENTED_EDGE('',*,*,#3422,.T.);
#4559=ORIENTED_EDGE('',*,*,#3423,.T.);
#4560=ORIENTED_EDGE('',*,*,#3424,.T.);
#4561=ORIENTED_EDGE('',*,*,#3425,.T.);
#4562=ORIENTED_EDGE('',*,*,#3426,.T.);
#4563=ORIENTED_EDGE('',*,*,#3427,.T.);
#4564=ORIENTED_EDGE('',*,*,#3428,.T.);
#4565=ORIENTED_EDGE('',*,*,#3429,.T.);
#4566=ORIENTED_EDGE('',*,*,#3430,.T.);
#4567=ORIENTED_EDGE('',*,*,#3431,.T.);
#4568=ORIENTED_EDGE('',*,*,#3432,.T.);
#4569=ORIENTED_EDGE('',*,*,#3433,.T.);
#4570=ORIENTED_EDGE('',*,*,#3434,.T.);
#4571=ORIENTED_EDGE('',*,*,#3435,.T.);
#4572=ORIENTED_EDGE('',*,*,#3436,.T.);
#4573=ORIENTED_EDGE('',*,*,#3437,.T.);
#4574=ORIENTED_EDGE('',*,*,#3438,.T.);
#4575=ORIENTED_EDGE('',*,*,#3439,.T.);
#4576=ORIENTED_EDGE('',*,*,#3440,.T.);
#4577=ORIENTED_EDGE('',*,*,#3441,.T.);
#4578=ORIENTED_EDGE('',*,*,#3442,.T.);
#4579=ORIENTED_EDGE('',*,*,#3250,.F.);
#4580=ORIENTED_EDGE('',*,*,#3443,.T.);
#4581=ORIENTED_EDGE('',*,*,#3362,.T.);
#4582=ORIENTED_EDGE('',*,*,#3443,.F.);
#4583=ORIENTED_EDGE('',*,*,#3444,.F.);
#4584=ORIENTED_EDGE('',*,*,#3363,.F.);
#4585=ORIENTED_EDGE('',*,*,#3445,.F.);
#4586=ORIENTED_EDGE('',*,*,#3280,.F.);
#4587=ORIENTED_EDGE('',*,*,#3445,.T.);
#4588=ORIENTED_EDGE('',*,*,#3442,.F.);
#4589=ORIENTED_EDGE('',*,*,#3446,.T.);
#4590=ORIENTED_EDGE('',*,*,#3281,.T.);
#4591=ORIENTED_EDGE('',*,*,#3446,.F.);
#4592=ORIENTED_EDGE('',*,*,#3441,.F.);
#4593=ORIENTED_EDGE('',*,*,#3447,.F.);
#4594=ORIENTED_EDGE('',*,*,#3282,.F.);
#4595=ORIENTED_EDGE('',*,*,#3447,.T.);
#4596=ORIENTED_EDGE('',*,*,#3440,.F.);
#4597=ORIENTED_EDGE('',*,*,#3448,.T.);
#4598=ORIENTED_EDGE('',*,*,#3283,.T.);
#4599=ORIENTED_EDGE('',*,*,#3448,.F.);
#4600=ORIENTED_EDGE('',*,*,#3439,.F.);
#4601=ORIENTED_EDGE('',*,*,#3449,.F.);
#4602=ORIENTED_EDGE('',*,*,#3284,.F.);
#4603=ORIENTED_EDGE('',*,*,#3449,.T.);
#4604=ORIENTED_EDGE('',*,*,#3438,.F.);
#4605=ORIENTED_EDGE('',*,*,#3450,.T.);
#4606=ORIENTED_EDGE('',*,*,#3285,.T.);
#4607=ORIENTED_EDGE('',*,*,#3450,.F.);
#4608=ORIENTED_EDGE('',*,*,#3437,.F.);
#4609=ORIENTED_EDGE('',*,*,#3451,.F.);
#4610=ORIENTED_EDGE('',*,*,#3286,.F.);
#4611=ORIENTED_EDGE('',*,*,#3451,.T.);
#4612=ORIENTED_EDGE('',*,*,#3436,.F.);
#4613=ORIENTED_EDGE('',*,*,#3452,.T.);
#4614=ORIENTED_EDGE('',*,*,#3287,.T.);
#4615=ORIENTED_EDGE('',*,*,#3452,.F.);
#4616=ORIENTED_EDGE('',*,*,#3435,.F.);
#4617=ORIENTED_EDGE('',*,*,#3453,.F.);
#4618=ORIENTED_EDGE('',*,*,#3288,.F.);
#4619=ORIENTED_EDGE('',*,*,#3453,.T.);
#4620=ORIENTED_EDGE('',*,*,#3434,.F.);
#4621=ORIENTED_EDGE('',*,*,#3454,.T.);
#4622=ORIENTED_EDGE('',*,*,#3289,.T.);
#4623=ORIENTED_EDGE('',*,*,#3454,.F.);
#4624=ORIENTED_EDGE('',*,*,#3433,.F.);
#4625=ORIENTED_EDGE('',*,*,#3455,.F.);
#4626=ORIENTED_EDGE('',*,*,#3290,.F.);
#4627=ORIENTED_EDGE('',*,*,#3455,.T.);
#4628=ORIENTED_EDGE('',*,*,#3432,.F.);
#4629=ORIENTED_EDGE('',*,*,#3456,.T.);
#4630=ORIENTED_EDGE('',*,*,#3291,.T.);
#4631=ORIENTED_EDGE('',*,*,#3456,.F.);
#4632=ORIENTED_EDGE('',*,*,#3431,.F.);
#4633=ORIENTED_EDGE('',*,*,#3457,.F.);
#4634=ORIENTED_EDGE('',*,*,#3292,.F.);
#4635=ORIENTED_EDGE('',*,*,#3457,.T.);
#4636=ORIENTED_EDGE('',*,*,#3430,.F.);
#4637=ORIENTED_EDGE('',*,*,#3458,.T.);
#4638=ORIENTED_EDGE('',*,*,#3293,.T.);
#4639=ORIENTED_EDGE('',*,*,#3458,.F.);
#4640=ORIENTED_EDGE('',*,*,#3429,.F.);
#4641=ORIENTED_EDGE('',*,*,#3459,.F.);
#4642=ORIENTED_EDGE('',*,*,#3294,.F.);
#4643=ORIENTED_EDGE('',*,*,#3459,.T.);
#4644=ORIENTED_EDGE('',*,*,#3428,.F.);
#4645=ORIENTED_EDGE('',*,*,#3460,.T.);
#4646=ORIENTED_EDGE('',*,*,#3295,.T.);
#4647=ORIENTED_EDGE('',*,*,#3460,.F.);
#4648=ORIENTED_EDGE('',*,*,#3427,.F.);
#4649=ORIENTED_EDGE('',*,*,#3461,.F.);
#4650=ORIENTED_EDGE('',*,*,#3296,.F.);
#4651=ORIENTED_EDGE('',*,*,#3461,.T.);
#4652=ORIENTED_EDGE('',*,*,#3426,.F.);
#4653=ORIENTED_EDGE('',*,*,#3462,.T.);
#4654=ORIENTED_EDGE('',*,*,#3297,.T.);
#4655=ORIENTED_EDGE('',*,*,#3462,.F.);
#4656=ORIENTED_EDGE('',*,*,#3425,.F.);
#4657=ORIENTED_EDGE('',*,*,#3463,.F.);
#4658=ORIENTED_EDGE('',*,*,#3298,.F.);
#4659=ORIENTED_EDGE('',*,*,#3463,.T.);
#4660=ORIENTED_EDGE('',*,*,#3424,.F.);
#4661=ORIENTED_EDGE('',*,*,#3464,.T.);
#4662=ORIENTED_EDGE('',*,*,#3299,.T.);
#4663=ORIENTED_EDGE('',*,*,#3464,.F.);
#4664=ORIENTED_EDGE('',*,*,#3423,.F.);
#4665=ORIENTED_EDGE('',*,*,#3465,.F.);
#4666=ORIENTED_EDGE('',*,*,#3300,.F.);
#4667=ORIENTED_EDGE('',*,*,#3465,.T.);
#4668=ORIENTED_EDGE('',*,*,#3422,.F.);
#4669=ORIENTED_EDGE('',*,*,#3466,.T.);
#4670=ORIENTED_EDGE('',*,*,#3301,.T.);
#4671=ORIENTED_EDGE('',*,*,#3466,.F.);
#4672=ORIENTED_EDGE('',*,*,#3421,.F.);
#4673=ORIENTED_EDGE('',*,*,#3467,.F.);
#4674=ORIENTED_EDGE('',*,*,#3302,.F.);
#4675=ORIENTED_EDGE('',*,*,#3467,.T.);
#4676=ORIENTED_EDGE('',*,*,#3420,.F.);
#4677=ORIENTED_EDGE('',*,*,#3468,.T.);
#4678=ORIENTED_EDGE('',*,*,#3303,.T.);
#4679=ORIENTED_EDGE('',*,*,#3468,.F.);
#4680=ORIENTED_EDGE('',*,*,#3419,.F.);
#4681=ORIENTED_EDGE('',*,*,#3469,.F.);
#4682=ORIENTED_EDGE('',*,*,#3304,.F.);
#4683=ORIENTED_EDGE('',*,*,#3469,.T.);
#4684=ORIENTED_EDGE('',*,*,#3418,.F.);
#4685=ORIENTED_EDGE('',*,*,#3470,.T.);
#4686=ORIENTED_EDGE('',*,*,#3305,.T.);
#4687=ORIENTED_EDGE('',*,*,#3470,.F.);
#4688=ORIENTED_EDGE('',*,*,#3417,.F.);
#4689=ORIENTED_EDGE('',*,*,#3471,.F.);
#4690=ORIENTED_EDGE('',*,*,#3306,.F.);
#4691=ORIENTED_EDGE('',*,*,#3471,.T.);
#4692=ORIENTED_EDGE('',*,*,#3416,.F.);
#4693=ORIENTED_EDGE('',*,*,#3472,.T.);
#4694=ORIENTED_EDGE('',*,*,#3307,.T.);
#4695=ORIENTED_EDGE('',*,*,#3472,.F.);
#4696=ORIENTED_EDGE('',*,*,#3415,.F.);
#4697=ORIENTED_EDGE('',*,*,#3473,.F.);
#4698=ORIENTED_EDGE('',*,*,#3308,.F.);
#4699=ORIENTED_EDGE('',*,*,#3473,.T.);
#4700=ORIENTED_EDGE('',*,*,#3414,.F.);
#4701=ORIENTED_EDGE('',*,*,#3474,.T.);
#4702=ORIENTED_EDGE('',*,*,#3309,.T.);
#4703=ORIENTED_EDGE('',*,*,#3474,.F.);
#4704=ORIENTED_EDGE('',*,*,#3413,.F.);
#4705=ORIENTED_EDGE('',*,*,#3475,.F.);
#4706=ORIENTED_EDGE('',*,*,#3310,.F.);
#4707=ORIENTED_EDGE('',*,*,#3475,.T.);
#4708=ORIENTED_EDGE('',*,*,#3412,.F.);
#4709=ORIENTED_EDGE('',*,*,#3476,.T.);
#4710=ORIENTED_EDGE('',*,*,#3311,.T.);
#4711=ORIENTED_EDGE('',*,*,#3476,.F.);
#4712=ORIENTED_EDGE('',*,*,#3411,.F.);
#4713=ORIENTED_EDGE('',*,*,#3477,.F.);
#4714=ORIENTED_EDGE('',*,*,#3312,.F.);
#4715=ORIENTED_EDGE('',*,*,#3477,.T.);
#4716=ORIENTED_EDGE('',*,*,#3410,.F.);
#4717=ORIENTED_EDGE('',*,*,#3478,.T.);
#4718=ORIENTED_EDGE('',*,*,#3313,.T.);
#4719=ORIENTED_EDGE('',*,*,#3478,.F.);
#4720=ORIENTED_EDGE('',*,*,#3409,.F.);
#4721=ORIENTED_EDGE('',*,*,#3479,.F.);
#4722=ORIENTED_EDGE('',*,*,#3314,.F.);
#4723=ORIENTED_EDGE('',*,*,#3479,.T.);
#4724=ORIENTED_EDGE('',*,*,#3408,.F.);
#4725=ORIENTED_EDGE('',*,*,#3480,.T.);
#4726=ORIENTED_EDGE('',*,*,#3315,.T.);
#4727=ORIENTED_EDGE('',*,*,#3480,.F.);
#4728=ORIENTED_EDGE('',*,*,#3407,.F.);
#4729=ORIENTED_EDGE('',*,*,#3481,.F.);
#4730=ORIENTED_EDGE('',*,*,#3316,.F.);
#4731=ORIENTED_EDGE('',*,*,#3481,.T.);
#4732=ORIENTED_EDGE('',*,*,#3406,.F.);
#4733=ORIENTED_EDGE('',*,*,#3482,.T.);
#4734=ORIENTED_EDGE('',*,*,#3317,.T.);
#4735=ORIENTED_EDGE('',*,*,#3482,.F.);
#4736=ORIENTED_EDGE('',*,*,#3405,.F.);
#4737=ORIENTED_EDGE('',*,*,#3483,.F.);
#4738=ORIENTED_EDGE('',*,*,#3318,.F.);
#4739=ORIENTED_EDGE('',*,*,#3483,.T.);
#4740=ORIENTED_EDGE('',*,*,#3404,.F.);
#4741=ORIENTED_EDGE('',*,*,#3484,.T.);
#4742=ORIENTED_EDGE('',*,*,#3319,.T.);
#4743=ORIENTED_EDGE('',*,*,#3484,.F.);
#4744=ORIENTED_EDGE('',*,*,#3403,.F.);
#4745=ORIENTED_EDGE('',*,*,#3485,.F.);
#4746=ORIENTED_EDGE('',*,*,#3320,.F.);
#4747=ORIENTED_EDGE('',*,*,#3485,.T.);
#4748=ORIENTED_EDGE('',*,*,#3402,.F.);
#4749=ORIENTED_EDGE('',*,*,#3486,.T.);
#4750=ORIENTED_EDGE('',*,*,#3321,.T.);
#4751=ORIENTED_EDGE('',*,*,#3486,.F.);
#4752=ORIENTED_EDGE('',*,*,#3401,.F.);
#4753=ORIENTED_EDGE('',*,*,#3487,.F.);
#4754=ORIENTED_EDGE('',*,*,#3322,.F.);
#4755=ORIENTED_EDGE('',*,*,#3487,.T.);
#4756=ORIENTED_EDGE('',*,*,#3400,.F.);
#4757=ORIENTED_EDGE('',*,*,#3488,.T.);
#4758=ORIENTED_EDGE('',*,*,#3323,.T.);
#4759=ORIENTED_EDGE('',*,*,#3488,.F.);
#4760=ORIENTED_EDGE('',*,*,#3399,.F.);
#4761=ORIENTED_EDGE('',*,*,#3489,.F.);
#4762=ORIENTED_EDGE('',*,*,#3324,.F.);
#4763=ORIENTED_EDGE('',*,*,#3489,.T.);
#4764=ORIENTED_EDGE('',*,*,#3398,.F.);
#4765=ORIENTED_EDGE('',*,*,#3490,.T.);
#4766=ORIENTED_EDGE('',*,*,#3325,.T.);
#4767=ORIENTED_EDGE('',*,*,#3490,.F.);
#4768=ORIENTED_EDGE('',*,*,#3397,.F.);
#4769=ORIENTED_EDGE('',*,*,#3491,.F.);
#4770=ORIENTED_EDGE('',*,*,#3326,.F.);
#4771=ORIENTED_EDGE('',*,*,#3491,.T.);
#4772=ORIENTED_EDGE('',*,*,#3396,.F.);
#4773=ORIENTED_EDGE('',*,*,#3492,.T.);
#4774=ORIENTED_EDGE('',*,*,#3327,.T.);
#4775=ORIENTED_EDGE('',*,*,#3492,.F.);
#4776=ORIENTED_EDGE('',*,*,#3395,.F.);
#4777=ORIENTED_EDGE('',*,*,#3493,.F.);
#4778=ORIENTED_EDGE('',*,*,#3328,.F.);
#4779=ORIENTED_EDGE('',*,*,#3493,.T.);
#4780=ORIENTED_EDGE('',*,*,#3394,.F.);
#4781=ORIENTED_EDGE('',*,*,#3494,.T.);
#4782=ORIENTED_EDGE('',*,*,#3329,.T.);
#4783=ORIENTED_EDGE('',*,*,#3494,.F.);
#4784=ORIENTED_EDGE('',*,*,#3393,.F.);
#4785=ORIENTED_EDGE('',*,*,#3495,.F.);
#4786=ORIENTED_EDGE('',*,*,#3330,.F.);
#4787=ORIENTED_EDGE('',*,*,#3495,.T.);
#4788=ORIENTED_EDGE('',*,*,#3392,.F.);
#4789=ORIENTED_EDGE('',*,*,#3496,.T.);
#4790=ORIENTED_EDGE('',*,*,#3331,.T.);
#4791=ORIENTED_EDGE('',*,*,#3496,.F.);
#4792=ORIENTED_EDGE('',*,*,#3391,.F.);
#4793=ORIENTED_EDGE('',*,*,#3497,.F.);
#4794=ORIENTED_EDGE('',*,*,#3332,.F.);
#4795=ORIENTED_EDGE('',*,*,#3497,.T.);
#4796=ORIENTED_EDGE('',*,*,#3390,.F.);
#4797=ORIENTED_EDGE('',*,*,#3498,.T.);
#4798=ORIENTED_EDGE('',*,*,#3333,.T.);
#4799=ORIENTED_EDGE('',*,*,#3498,.F.);
#4800=ORIENTED_EDGE('',*,*,#3389,.F.);
#4801=ORIENTED_EDGE('',*,*,#3499,.F.);
#4802=ORIENTED_EDGE('',*,*,#3334,.F.);
#4803=ORIENTED_EDGE('',*,*,#3499,.T.);
#4804=ORIENTED_EDGE('',*,*,#3388,.F.);
#4805=ORIENTED_EDGE('',*,*,#3500,.T.);
#4806=ORIENTED_EDGE('',*,*,#3335,.T.);
#4807=ORIENTED_EDGE('',*,*,#3500,.F.);
#4808=ORIENTED_EDGE('',*,*,#3387,.F.);
#4809=ORIENTED_EDGE('',*,*,#3501,.F.);
#4810=ORIENTED_EDGE('',*,*,#3336,.F.);
#4811=ORIENTED_EDGE('',*,*,#3501,.T.);
#4812=ORIENTED_EDGE('',*,*,#3386,.F.);
#4813=ORIENTED_EDGE('',*,*,#3502,.T.);
#4814=ORIENTED_EDGE('',*,*,#3337,.T.);
#4815=ORIENTED_EDGE('',*,*,#3502,.F.);
#4816=ORIENTED_EDGE('',*,*,#3385,.F.);
#4817=ORIENTED_EDGE('',*,*,#3503,.F.);
#4818=ORIENTED_EDGE('',*,*,#3338,.F.);
#4819=ORIENTED_EDGE('',*,*,#3503,.T.);
#4820=ORIENTED_EDGE('',*,*,#3384,.F.);
#4821=ORIENTED_EDGE('',*,*,#3504,.T.);
#4822=ORIENTED_EDGE('',*,*,#3339,.T.);
#4823=ORIENTED_EDGE('',*,*,#3504,.F.);
#4824=ORIENTED_EDGE('',*,*,#3383,.F.);
#4825=ORIENTED_EDGE('',*,*,#3505,.F.);
#4826=ORIENTED_EDGE('',*,*,#3340,.F.);
#4827=ORIENTED_EDGE('',*,*,#3505,.T.);
#4828=ORIENTED_EDGE('',*,*,#3382,.F.);
#4829=ORIENTED_EDGE('',*,*,#3506,.T.);
#4830=ORIENTED_EDGE('',*,*,#3341,.T.);
#4831=ORIENTED_EDGE('',*,*,#3506,.F.);
#4832=ORIENTED_EDGE('',*,*,#3381,.F.);
#4833=ORIENTED_EDGE('',*,*,#3507,.F.);
#4834=ORIENTED_EDGE('',*,*,#3342,.F.);
#4835=ORIENTED_EDGE('',*,*,#3507,.T.);
#4836=ORIENTED_EDGE('',*,*,#3380,.F.);
#4837=ORIENTED_EDGE('',*,*,#3508,.T.);
#4838=ORIENTED_EDGE('',*,*,#3343,.T.);
#4839=ORIENTED_EDGE('',*,*,#3508,.F.);
#4840=ORIENTED_EDGE('',*,*,#3379,.F.);
#4841=ORIENTED_EDGE('',*,*,#3509,.F.);
#4842=ORIENTED_EDGE('',*,*,#3344,.F.);
#4843=ORIENTED_EDGE('',*,*,#3509,.T.);
#4844=ORIENTED_EDGE('',*,*,#3378,.F.);
#4845=ORIENTED_EDGE('',*,*,#3510,.T.);
#4846=ORIENTED_EDGE('',*,*,#3345,.T.);
#4847=ORIENTED_EDGE('',*,*,#3510,.F.);
#4848=ORIENTED_EDGE('',*,*,#3377,.F.);
#4849=ORIENTED_EDGE('',*,*,#3511,.F.);
#4850=ORIENTED_EDGE('',*,*,#3346,.F.);
#4851=ORIENTED_EDGE('',*,*,#3511,.T.);
#4852=ORIENTED_EDGE('',*,*,#3376,.F.);
#4853=ORIENTED_EDGE('',*,*,#3512,.T.);
#4854=ORIENTED_EDGE('',*,*,#3347,.T.);
#4855=ORIENTED_EDGE('',*,*,#3512,.F.);
#4856=ORIENTED_EDGE('',*,*,#3375,.F.);
#4857=ORIENTED_EDGE('',*,*,#3513,.F.);
#4858=ORIENTED_EDGE('',*,*,#3348,.F.);
#4859=ORIENTED_EDGE('',*,*,#3513,.T.);
#4860=ORIENTED_EDGE('',*,*,#3374,.F.);
#4861=ORIENTED_EDGE('',*,*,#3514,.T.);
#4862=ORIENTED_EDGE('',*,*,#3349,.T.);
#4863=ORIENTED_EDGE('',*,*,#3514,.F.);
#4864=ORIENTED_EDGE('',*,*,#3373,.F.);
#4865=ORIENTED_EDGE('',*,*,#3515,.F.);
#4866=ORIENTED_EDGE('',*,*,#3350,.F.);
#4867=ORIENTED_EDGE('',*,*,#3515,.T.);
#4868=ORIENTED_EDGE('',*,*,#3372,.F.);
#4869=ORIENTED_EDGE('',*,*,#3516,.T.);
#4870=ORIENTED_EDGE('',*,*,#3351,.T.);
#4871=ORIENTED_EDGE('',*,*,#3516,.F.);
#4872=ORIENTED_EDGE('',*,*,#3371,.F.);
#4873=ORIENTED_EDGE('',*,*,#3517,.F.);
#4874=ORIENTED_EDGE('',*,*,#3352,.F.);
#4875=ORIENTED_EDGE('',*,*,#3517,.T.);
#4876=ORIENTED_EDGE('',*,*,#3370,.F.);
#4877=ORIENTED_EDGE('',*,*,#3518,.T.);
#4878=ORIENTED_EDGE('',*,*,#3353,.T.);
#4879=ORIENTED_EDGE('',*,*,#3518,.F.);
#4880=ORIENTED_EDGE('',*,*,#3369,.F.);
#4881=ORIENTED_EDGE('',*,*,#3519,.F.);
#4882=ORIENTED_EDGE('',*,*,#3354,.F.);
#4883=ORIENTED_EDGE('',*,*,#3519,.T.);
#4884=ORIENTED_EDGE('',*,*,#3368,.F.);
#4885=ORIENTED_EDGE('',*,*,#3520,.T.);
#4886=ORIENTED_EDGE('',*,*,#3355,.T.);
#4887=ORIENTED_EDGE('',*,*,#3521,.F.);
#4888=ORIENTED_EDGE('',*,*,#3356,.F.);
#4889=ORIENTED_EDGE('',*,*,#3520,.F.);
#4890=ORIENTED_EDGE('',*,*,#3367,.F.);
#4891=ORIENTED_EDGE('',*,*,#3444,.T.);
#4892=ORIENTED_EDGE('',*,*,#3359,.T.);
#4893=ORIENTED_EDGE('',*,*,#3522,.T.);
#4894=ORIENTED_EDGE('',*,*,#3364,.F.);
#4895=ORIENTED_EDGE('',*,*,#3523,.F.);
#4896=ORIENTED_EDGE('',*,*,#3365,.F.);
#4897=ORIENTED_EDGE('',*,*,#3522,.F.);
#4898=ORIENTED_EDGE('',*,*,#3358,.F.);
#4899=ORIENTED_EDGE('',*,*,#3521,.T.);
#4900=ORIENTED_EDGE('',*,*,#3366,.F.);
#4901=ORIENTED_EDGE('',*,*,#3523,.T.);
#4902=ORIENTED_EDGE('',*,*,#3357,.T.);
#5168=CYLINDRICAL_SURFACE('',#6215,0.6);
#5169=CYLINDRICAL_SURFACE('',#6217,0.125);
#5170=CYLINDRICAL_SURFACE('',#6218,0.125);
#5171=CYLINDRICAL_SURFACE('',#6219,1.);
#5172=CYLINDRICAL_SURFACE('',#6222,0.125);
#5173=CYLINDRICAL_SURFACE('',#6223,0.125);
#5174=CYLINDRICAL_SURFACE('',#6307,1.4);
#5175=CYLINDRICAL_SURFACE('',#6392,1.4);
#5176=CYLINDRICAL_SURFACE('',#6393,0.0555000000000001);
#5177=CYLINDRICAL_SURFACE('',#6394,1.24783954473516);
#5178=CYLINDRICAL_SURFACE('',#6395,0.0555000000000001);
#5179=CYLINDRICAL_SURFACE('',#6396,1.24783954473516);
#5180=CYLINDRICAL_SURFACE('',#6397,0.0555000000000001);
#5181=CYLINDRICAL_SURFACE('',#6398,1.24783954473516);
#5182=CYLINDRICAL_SURFACE('',#6399,0.0555000000000001);
#5183=CYLINDRICAL_SURFACE('',#6400,1.24783954473516);
#5184=CYLINDRICAL_SURFACE('',#6401,0.0555000000000001);
#5185=CYLINDRICAL_SURFACE('',#6402,1.24783954473516);
#5186=CYLINDRICAL_SURFACE('',#6403,0.0555000000000001);
#5187=CYLINDRICAL_SURFACE('',#6404,1.24783954473516);
#5188=CYLINDRICAL_SURFACE('',#6405,0.0555000000000001);
#5189=CYLINDRICAL_SURFACE('',#6406,1.24783954473516);
#5190=CYLINDRICAL_SURFACE('',#6407,0.0555000000000001);
#5191=CYLINDRICAL_SURFACE('',#6408,1.24783954473516);
#5192=CYLINDRICAL_SURFACE('',#6409,0.0555000000000001);
#5193=CYLINDRICAL_SURFACE('',#6410,1.24783954473516);
#5194=CYLINDRICAL_SURFACE('',#6411,0.0555000000000001);
#5195=CYLINDRICAL_SURFACE('',#6412,1.24783954473516);
#5196=CYLINDRICAL_SURFACE('',#6413,0.0555000000000001);
#5197=CYLINDRICAL_SURFACE('',#6414,1.24783954473516);
#5198=CYLINDRICAL_SURFACE('',#6415,0.0555000000000001);
#5199=CYLINDRICAL_SURFACE('',#6416,1.24783954473516);
#5200=CYLINDRICAL_SURFACE('',#6417,0.0555000000000001);
#5201=CYLINDRICAL_SURFACE('',#6418,1.24783954473516);
#5202=CYLINDRICAL_SURFACE('',#6419,0.0555000000000001);
#5203=CYLINDRICAL_SURFACE('',#6420,1.24783954473516);
#5204=CYLINDRICAL_SURFACE('',#6421,0.0555000000000001);
#5205=CYLINDRICAL_SURFACE('',#6422,1.24783954473516);
#5206=CYLINDRICAL_SURFACE('',#6423,0.0555000000000001);
#5207=CYLINDRICAL_SURFACE('',#6424,1.24783954473516);
#5208=CYLINDRICAL_SURFACE('',#6425,0.0555000000000001);
#5209=CYLINDRICAL_SURFACE('',#6426,1.24783954473516);
#5210=CYLINDRICAL_SURFACE('',#6427,0.0555000000000001);
#5211=CYLINDRICAL_SURFACE('',#6428,1.24783954473516);
#5212=CYLINDRICAL_SURFACE('',#6429,0.0555000000000001);
#5213=CYLINDRICAL_SURFACE('',#6430,1.24783954473516);
#5214=CYLINDRICAL_SURFACE('',#6431,0.0555000000000001);
#5215=CYLINDRICAL_SURFACE('',#6432,1.24783954473516);
#5216=CYLINDRICAL_SURFACE('',#6433,0.0555000000000001);
#5217=CYLINDRICAL_SURFACE('',#6434,1.24783954473516);
#5218=CYLINDRICAL_SURFACE('',#6435,0.0555000000000001);
#5219=CYLINDRICAL_SURFACE('',#6436,1.24783954473516);
#5220=CYLINDRICAL_SURFACE('',#6437,0.0555000000000001);
#5221=CYLINDRICAL_SURFACE('',#6438,1.24783954473516);
#5222=CYLINDRICAL_SURFACE('',#6439,0.0555000000000001);
#5223=CYLINDRICAL_SURFACE('',#6440,1.24783954473516);
#5224=CYLINDRICAL_SURFACE('',#6441,0.0555000000000001);
#5225=CYLINDRICAL_SURFACE('',#6442,1.24783954473516);
#5226=CYLINDRICAL_SURFACE('',#6443,0.0555000000000001);
#5227=CYLINDRICAL_SURFACE('',#6444,1.24783954473516);
#5228=CYLINDRICAL_SURFACE('',#6445,0.0555000000000001);
#5229=CYLINDRICAL_SURFACE('',#6446,1.24783954473516);
#5230=CYLINDRICAL_SURFACE('',#6447,0.0555000000000001);
#5231=CYLINDRICAL_SURFACE('',#6448,1.24783954473516);
#5232=CYLINDRICAL_SURFACE('',#6449,0.0555000000000001);
#5233=CYLINDRICAL_SURFACE('',#6450,1.24783954473516);
#5234=CYLINDRICAL_SURFACE('',#6451,0.0555000000000001);
#5235=CYLINDRICAL_SURFACE('',#6452,1.24783954473516);
#5236=CYLINDRICAL_SURFACE('',#6453,0.0555000000000001);
#5237=CYLINDRICAL_SURFACE('',#6454,1.24783954473516);
#5238=CYLINDRICAL_SURFACE('',#6455,0.0555000000000001);
#5239=CYLINDRICAL_SURFACE('',#6456,1.24783954473516);
#5240=CYLINDRICAL_SURFACE('',#6457,0.0555000000000001);
#5241=CYLINDRICAL_SURFACE('',#6458,1.24783954473516);
#5242=CYLINDRICAL_SURFACE('',#6459,0.0555000000000001);
#5243=CYLINDRICAL_SURFACE('',#6460,1.24783954473516);
#5244=CYLINDRICAL_SURFACE('',#6461,0.0555000000000001);
#5245=CYLINDRICAL_SURFACE('',#6462,1.24783954473516);
#5246=CYLINDRICAL_SURFACE('',#6463,0.0555000000000001);
#5247=CYLINDRICAL_SURFACE('',#6464,1.24783954473516);
#5248=CYLINDRICAL_SURFACE('',#6465,0.0555000000000001);
#5249=CYLINDRICAL_SURFACE('',#6466,1.24783954473516);
#5250=CYLINDRICAL_SURFACE('',#6467,0.0555000000000001);
#5251=CYLINDRICAL_SURFACE('',#6468,1.24783954473516);
#5252=CYLINDRICAL_SURFACE('',#6469,0.0555000000000001);
#5253=CYLINDRICAL_SURFACE('',#6470,1.24783954473516);
#5254=CYLINDRICAL_SURFACE('',#6471,0.0555000000000001);
#5255=CYLINDRICAL_SURFACE('',#6472,1.24783954473516);
#5428=ADVANCED_FACE('',(#757),#540,.F.);
#5429=ADVANCED_FACE('',(#758,#417),#541,.F.);
#5430=ADVANCED_FACE('',(#759),#542,.F.);
#5431=ADVANCED_FACE('',(#760,#418),#543,.T.);
#5432=ADVANCED_FACE('',(#761,#419,#420,#421),#5168,.F.);
#5433=ADVANCED_FACE('',(#762),#5169,.F.);
#5434=ADVANCED_FACE('',(#763),#5170,.F.);
#5435=ADVANCED_FACE('',(#764,#422,#423,#424),#5171,.T.);
#5436=ADVANCED_FACE('',(#765),#5172,.F.);
#5437=ADVANCED_FACE('',(#766),#5173,.F.);
#5438=ADVANCED_FACE('',(#767,#425),#544,.F.);
#5439=ADVANCED_FACE('',(#768,#426),#545,.T.);
#5440=ADVANCED_FACE('',(#769),#5174,.T.);
#5441=ADVANCED_FACE('',(#770,#427),#546,.F.);
#5442=ADVANCED_FACE('',(#771,#428),#547,.F.);
#5443=ADVANCED_FACE('',(#772),#5175,.T.);
#5444=ADVANCED_FACE('',(#773),#5176,.F.);
#5445=ADVANCED_FACE('',(#774),#5177,.T.);
#5446=ADVANCED_FACE('',(#775),#5178,.F.);
#5447=ADVANCED_FACE('',(#776),#5179,.T.);
#5448=ADVANCED_FACE('',(#777),#5180,.F.);
#5449=ADVANCED_FACE('',(#778),#5181,.T.);
#5450=ADVANCED_FACE('',(#779),#5182,.F.);
#5451=ADVANCED_FACE('',(#780),#5183,.T.);
#5452=ADVANCED_FACE('',(#781),#5184,.F.);
#5453=ADVANCED_FACE('',(#782),#5185,.T.);
#5454=ADVANCED_FACE('',(#783),#5186,.F.);
#5455=ADVANCED_FACE('',(#784),#5187,.T.);
#5456=ADVANCED_FACE('',(#785),#5188,.F.);
#5457=ADVANCED_FACE('',(#786),#5189,.T.);
#5458=ADVANCED_FACE('',(#787),#5190,.F.);
#5459=ADVANCED_FACE('',(#788),#5191,.T.);
#5460=ADVANCED_FACE('',(#789),#5192,.F.);
#5461=ADVANCED_FACE('',(#790),#5193,.T.);
#5462=ADVANCED_FACE('',(#791),#5194,.F.);
#5463=ADVANCED_FACE('',(#792),#5195,.T.);
#5464=ADVANCED_FACE('',(#793),#5196,.F.);
#5465=ADVANCED_FACE('',(#794),#5197,.T.);
#5466=ADVANCED_FACE('',(#795),#5198,.F.);
#5467=ADVANCED_FACE('',(#796),#5199,.T.);
#5468=ADVANCED_FACE('',(#797),#5200,.F.);
#5469=ADVANCED_FACE('',(#798),#5201,.T.);
#5470=ADVANCED_FACE('',(#799),#5202,.F.);
#5471=ADVANCED_FACE('',(#800),#5203,.T.);
#5472=ADVANCED_FACE('',(#801),#5204,.F.);
#5473=ADVANCED_FACE('',(#802),#5205,.T.);
#5474=ADVANCED_FACE('',(#803),#5206,.F.);
#5475=ADVANCED_FACE('',(#804),#5207,.T.);
#5476=ADVANCED_FACE('',(#805),#5208,.F.);
#5477=ADVANCED_FACE('',(#806),#5209,.T.);
#5478=ADVANCED_FACE('',(#807),#5210,.F.);
#5479=ADVANCED_FACE('',(#808),#5211,.T.);
#5480=ADVANCED_FACE('',(#809),#5212,.F.);
#5481=ADVANCED_FACE('',(#810),#5213,.T.);
#5482=ADVANCED_FACE('',(#811),#5214,.F.);
#5483=ADVANCED_FACE('',(#812),#5215,.T.);
#5484=ADVANCED_FACE('',(#813),#5216,.F.);
#5485=ADVANCED_FACE('',(#814),#5217,.T.);
#5486=ADVANCED_FACE('',(#815),#5218,.F.);
#5487=ADVANCED_FACE('',(#816),#5219,.T.);
#5488=ADVANCED_FACE('',(#817),#5220,.F.);
#5489=ADVANCED_FACE('',(#818),#5221,.T.);
#5490=ADVANCED_FACE('',(#819),#5222,.F.);
#5491=ADVANCED_FACE('',(#820),#5223,.T.);
#5492=ADVANCED_FACE('',(#821),#5224,.F.);
#5493=ADVANCED_FACE('',(#822),#5225,.T.);
#5494=ADVANCED_FACE('',(#823),#5226,.F.);
#5495=ADVANCED_FACE('',(#824),#5227,.T.);
#5496=ADVANCED_FACE('',(#825),#5228,.F.);
#5497=ADVANCED_FACE('',(#826),#5229,.T.);
#5498=ADVANCED_FACE('',(#827),#5230,.F.);
#5499=ADVANCED_FACE('',(#828),#5231,.T.);
#5500=ADVANCED_FACE('',(#829),#5232,.F.);
#5501=ADVANCED_FACE('',(#830),#5233,.T.);
#5502=ADVANCED_FACE('',(#831),#5234,.F.);
#5503=ADVANCED_FACE('',(#832),#5235,.T.);
#5504=ADVANCED_FACE('',(#833),#5236,.F.);
#5505=ADVANCED_FACE('',(#834),#5237,.T.);
#5506=ADVANCED_FACE('',(#835),#5238,.F.);
#5507=ADVANCED_FACE('',(#836),#5239,.T.);
#5508=ADVANCED_FACE('',(#837),#5240,.F.);
#5509=ADVANCED_FACE('',(#838),#5241,.T.);
#5510=ADVANCED_FACE('',(#839),#5242,.F.);
#5511=ADVANCED_FACE('',(#840),#5243,.T.);
#5512=ADVANCED_FACE('',(#841),#5244,.F.);
#5513=ADVANCED_FACE('',(#842),#5245,.T.);
#5514=ADVANCED_FACE('',(#843),#5246,.F.);
#5515=ADVANCED_FACE('',(#844),#5247,.T.);
#5516=ADVANCED_FACE('',(#845),#5248,.F.);
#5517=ADVANCED_FACE('',(#846),#5249,.T.);
#5518=ADVANCED_FACE('',(#847),#5250,.F.);
#5519=ADVANCED_FACE('',(#848),#5251,.T.);
#5520=ADVANCED_FACE('',(#849),#5252,.F.);
#5521=ADVANCED_FACE('',(#850),#5253,.T.);
#5522=ADVANCED_FACE('',(#851),#5254,.F.);
#5523=ADVANCED_FACE('',(#852),#5255,.T.);
#5595=CLOSED_SHELL('',(#5428,#5429,#5430,#5431,#5432,#5433,#5434,#5435,
#5436,#5437,#5438,#5439,#5440,#5441,#5442,#5443,#5444,#5445,#5446,#5447,
#5448,#5449,#5450,#5451,#5452,#5453,#5454,#5455,#5456,#5457,#5458,#5459,
#5460,#5461,#5462,#5463,#5464,#5465,#5466,#5467,#5468,#5469,#5470,#5471,
#5472,#5473,#5474,#5475,#5476,#5477,#5478,#5479,#5480,#5481,#5482,#5483,
#5484,#5485,#5486,#5487,#5488,#5489,#5490,#5491,#5492,#5493,#5494,#5495,
#5496,#5497,#5498,#5499,#5500,#5501,#5502,#5503,#5504,#5505,#5506,#5507,
#5508,#5509,#5510,#5511,#5512,#5513,#5514,#5515,#5516,#5517,#5518,#5519,
#5520,#5521,#5522,#5523));
#6207=AXIS2_PLACEMENT_3D('',#9698,#7417,#7418);
#6208=AXIS2_PLACEMENT_3D('',#9699,#7419,#7420);
#6209=AXIS2_PLACEMENT_3D('',#9708,#7425,#7426);
#6210=AXIS2_PLACEMENT_3D('',#9715,#7430,#7431);
#6211=AXIS2_PLACEMENT_3D('',#9716,#7432,#7433);
#6212=AXIS2_PLACEMENT_3D('',#9722,#7437,#7438);
#6213=AXIS2_PLACEMENT_3D('',#9724,#7439,#7440);
#6214=AXIS2_PLACEMENT_3D('',#9725,#7441,#7442);
#6215=AXIS2_PLACEMENT_3D('',#9726,#7443,#7444);
#6216=AXIS2_PLACEMENT_3D('',#9727,#7445,#7446);
#6217=AXIS2_PLACEMENT_3D('',#9842,#7447,#7448);
#6218=AXIS2_PLACEMENT_3D('',#9885,#7450,#7451);
#6219=AXIS2_PLACEMENT_3D('',#9928,#7453,#7454);
#6220=AXIS2_PLACEMENT_3D('',#9930,#7455,#7456);
#6221=AXIS2_PLACEMENT_3D('',#9934,#7459,#7460);
#6222=AXIS2_PLACEMENT_3D('',#10017,#7461,#7462);
#6223=AXIS2_PLACEMENT_3D('',#10019,#7464,#7465);
#6224=AXIS2_PLACEMENT_3D('',#10021,#7467,#7468);
#6225=AXIS2_PLACEMENT_3D('',#10022,#7469,#7470);
#6226=AXIS2_PLACEMENT_3D('',#10024,#7471,#7472);
#6227=AXIS2_PLACEMENT_3D('',#10027,#7473,#7474);
#6228=AXIS2_PLACEMENT_3D('',#10029,#7475,#7476);
#6229=AXIS2_PLACEMENT_3D('',#10031,#7477,#7478);
#6230=AXIS2_PLACEMENT_3D('',#10033,#7479,#7480);
#6231=AXIS2_PLACEMENT_3D('',#10035,#7481,#7482);
#6232=AXIS2_PLACEMENT_3D('',#10037,#7483,#7484);
#6233=AXIS2_PLACEMENT_3D('',#10039,#7485,#7486);
#6234=AXIS2_PLACEMENT_3D('',#10041,#7487,#7488);
#6235=AXIS2_PLACEMENT_3D('',#10043,#7489,#7490);
#6236=AXIS2_PLACEMENT_3D('',#10045,#7491,#7492);
#6237=AXIS2_PLACEMENT_3D('',#10047,#7493,#7494);
#6238=AXIS2_PLACEMENT_3D('',#10049,#7495,#7496);
#6239=AXIS2_PLACEMENT_3D('',#10051,#7497,#7498);
#6240=AXIS2_PLACEMENT_3D('',#10053,#7499,#7500);
#6241=AXIS2_PLACEMENT_3D('',#10055,#7501,#7502);
#6242=AXIS2_PLACEMENT_3D('',#10057,#7503,#7504);
#6243=AXIS2_PLACEMENT_3D('',#10059,#7505,#7506);
#6244=AXIS2_PLACEMENT_3D('',#10061,#7507,#7508);
#6245=AXIS2_PLACEMENT_3D('',#10063,#7509,#7510);
#6246=AXIS2_PLACEMENT_3D('',#10065,#7511,#7512);
#6247=AXIS2_PLACEMENT_3D('',#10067,#7513,#7514);
#6248=AXIS2_PLACEMENT_3D('',#10069,#7515,#7516);
#6249=AXIS2_PLACEMENT_3D('',#10071,#7517,#7518);
#6250=AXIS2_PLACEMENT_3D('',#10073,#7519,#7520);
#6251=AXIS2_PLACEMENT_3D('',#10075,#7521,#7522);
#6252=AXIS2_PLACEMENT_3D('',#10077,#7523,#7524);
#6253=AXIS2_PLACEMENT_3D('',#10079,#7525,#7526);
#6254=AXIS2_PLACEMENT_3D('',#10081,#7527,#7528);
#6255=AXIS2_PLACEMENT_3D('',#10083,#7529,#7530);
#6256=AXIS2_PLACEMENT_3D('',#10085,#7531,#7532);
#6257=AXIS2_PLACEMENT_3D('',#10087,#7533,#7534);
#6258=AXIS2_PLACEMENT_3D('',#10089,#7535,#7536);
#6259=AXIS2_PLACEMENT_3D('',#10091,#7537,#7538);
#6260=AXIS2_PLACEMENT_3D('',#10093,#7539,#7540);
#6261=AXIS2_PLACEMENT_3D('',#10095,#7541,#7542);
#6262=AXIS2_PLACEMENT_3D('',#10097,#7543,#7544);
#6263=AXIS2_PLACEMENT_3D('',#10099,#7545,#7546);
#6264=AXIS2_PLACEMENT_3D('',#10101,#7547,#7548);
#6265=AXIS2_PLACEMENT_3D('',#10103,#7549,#7550);
#6266=AXIS2_PLACEMENT_3D('',#10105,#7551,#7552);
#6267=AXIS2_PLACEMENT_3D('',#10107,#7553,#7554);
#6268=AXIS2_PLACEMENT_3D('',#10109,#7555,#7556);
#6269=AXIS2_PLACEMENT_3D('',#10111,#7557,#7558);
#6270=AXIS2_PLACEMENT_3D('',#10113,#7559,#7560);
#6271=AXIS2_PLACEMENT_3D('',#10115,#7561,#7562);
#6272=AXIS2_PLACEMENT_3D('',#10117,#7563,#7564);
#6273=AXIS2_PLACEMENT_3D('',#10119,#7565,#7566);
#6274=AXIS2_PLACEMENT_3D('',#10121,#7567,#7568);
#6275=AXIS2_PLACEMENT_3D('',#10123,#7569,#7570);
#6276=AXIS2_PLACEMENT_3D('',#10125,#7571,#7572);
#6277=AXIS2_PLACEMENT_3D('',#10127,#7573,#7574);
#6278=AXIS2_PLACEMENT_3D('',#10129,#7575,#7576);
#6279=AXIS2_PLACEMENT_3D('',#10131,#7577,#7578);
#6280=AXIS2_PLACEMENT_3D('',#10133,#7579,#7580);
#6281=AXIS2_PLACEMENT_3D('',#10135,#7581,#7582);
#6282=AXIS2_PLACEMENT_3D('',#10137,#7583,#7584);
#6283=AXIS2_PLACEMENT_3D('',#10139,#7585,#7586);
#6284=AXIS2_PLACEMENT_3D('',#10141,#7587,#7588);
#6285=AXIS2_PLACEMENT_3D('',#10143,#7589,#7590);
#6286=AXIS2_PLACEMENT_3D('',#10145,#7591,#7592);
#6287=AXIS2_PLACEMENT_3D('',#10147,#7593,#7594);
#6288=AXIS2_PLACEMENT_3D('',#10149,#7595,#7596);
#6289=AXIS2_PLACEMENT_3D('',#10151,#7597,#7598);
#6290=AXIS2_PLACEMENT_3D('',#10153,#7599,#7600);
#6291=AXIS2_PLACEMENT_3D('',#10155,#7601,#7602);
#6292=AXIS2_PLACEMENT_3D('',#10157,#7603,#7604);
#6293=AXIS2_PLACEMENT_3D('',#10159,#7605,#7606);
#6294=AXIS2_PLACEMENT_3D('',#10161,#7607,#7608);
#6295=AXIS2_PLACEMENT_3D('',#10163,#7609,#7610);
#6296=AXIS2_PLACEMENT_3D('',#10165,#7611,#7612);
#6297=AXIS2_PLACEMENT_3D('',#10167,#7613,#7614);
#6298=AXIS2_PLACEMENT_3D('',#10169,#7615,#7616);
#6299=AXIS2_PLACEMENT_3D('',#10171,#7617,#7618);
#6300=AXIS2_PLACEMENT_3D('',#10173,#7619,#7620);
#6301=AXIS2_PLACEMENT_3D('',#10175,#7621,#7622);
#6302=AXIS2_PLACEMENT_3D('',#10177,#7623,#7624);
#6303=AXIS2_PLACEMENT_3D('',#10179,#7625,#7626);
#6304=AXIS2_PLACEMENT_3D('',#10181,#7627,#7628);
#6305=AXIS2_PLACEMENT_3D('',#10183,#7629,#7630);
#6306=AXIS2_PLACEMENT_3D('',#10184,#7631,#7632);
#6307=AXIS2_PLACEMENT_3D('',#10185,#7633,#7634);
#6308=AXIS2_PLACEMENT_3D('',#10187,#7635,#7636);
#6309=AXIS2_PLACEMENT_3D('',#10189,#7638,#7639);
#6310=AXIS2_PLACEMENT_3D('',#10190,#7640,#7641);
#6311=AXIS2_PLACEMENT_3D('',#10192,#7642,#7643);
#6312=AXIS2_PLACEMENT_3D('',#10195,#7644,#7645);
#6313=AXIS2_PLACEMENT_3D('',#10197,#7646,#7647);
#6314=AXIS2_PLACEMENT_3D('',#10199,#7648,#7649);
#6315=AXIS2_PLACEMENT_3D('',#10201,#7650,#7651);
#6316=AXIS2_PLACEMENT_3D('',#10203,#7652,#7653);
#6317=AXIS2_PLACEMENT_3D('',#10205,#7654,#7655);
#6318=AXIS2_PLACEMENT_3D('',#10207,#7656,#7657);
#6319=AXIS2_PLACEMENT_3D('',#10209,#7658,#7659);
#6320=AXIS2_PLACEMENT_3D('',#10211,#7660,#7661);
#6321=AXIS2_PLACEMENT_3D('',#10213,#7662,#7663);
#6322=AXIS2_PLACEMENT_3D('',#10215,#7664,#7665);
#6323=AXIS2_PLACEMENT_3D('',#10217,#7666,#7667);
#6324=AXIS2_PLACEMENT_3D('',#10219,#7668,#7669);
#6325=AXIS2_PLACEMENT_3D('',#10221,#7670,#7671);
#6326=AXIS2_PLACEMENT_3D('',#10223,#7672,#7673);
#6327=AXIS2_PLACEMENT_3D('',#10225,#7674,#7675);
#6328=AXIS2_PLACEMENT_3D('',#10227,#7676,#7677);
#6329=AXIS2_PLACEMENT_3D('',#10229,#7678,#7679);
#6330=AXIS2_PLACEMENT_3D('',#10231,#7680,#7681);
#6331=AXIS2_PLACEMENT_3D('',#10233,#7682,#7683);
#6332=AXIS2_PLACEMENT_3D('',#10235,#7684,#7685);
#6333=AXIS2_PLACEMENT_3D('',#10237,#7686,#7687);
#6334=AXIS2_PLACEMENT_3D('',#10239,#7688,#7689);
#6335=AXIS2_PLACEMENT_3D('',#10241,#7690,#7691);
#6336=AXIS2_PLACEMENT_3D('',#10243,#7692,#7693);
#6337=AXIS2_PLACEMENT_3D('',#10245,#7694,#7695);
#6338=AXIS2_PLACEMENT_3D('',#10247,#7696,#7697);
#6339=AXIS2_PLACEMENT_3D('',#10249,#7698,#7699);
#6340=AXIS2_PLACEMENT_3D('',#10251,#7700,#7701);
#6341=AXIS2_PLACEMENT_3D('',#10253,#7702,#7703);
#6342=AXIS2_PLACEMENT_3D('',#10255,#7704,#7705);
#6343=AXIS2_PLACEMENT_3D('',#10257,#7706,#7707);
#6344=AXIS2_PLACEMENT_3D('',#10259,#7708,#7709);
#6345=AXIS2_PLACEMENT_3D('',#10261,#7710,#7711);
#6346=AXIS2_PLACEMENT_3D('',#10263,#7712,#7713);
#6347=AXIS2_PLACEMENT_3D('',#10265,#7714,#7715);
#6348=AXIS2_PLACEMENT_3D('',#10267,#7716,#7717);
#6349=AXIS2_PLACEMENT_3D('',#10269,#7718,#7719);
#6350=AXIS2_PLACEMENT_3D('',#10271,#7720,#7721);
#6351=AXIS2_PLACEMENT_3D('',#10273,#7722,#7723);
#6352=AXIS2_PLACEMENT_3D('',#10275,#7724,#7725);
#6353=AXIS2_PLACEMENT_3D('',#10277,#7726,#7727);
#6354=AXIS2_PLACEMENT_3D('',#10279,#7728,#7729);
#6355=AXIS2_PLACEMENT_3D('',#10281,#7730,#7731);
#6356=AXIS2_PLACEMENT_3D('',#10283,#7732,#7733);
#6357=AXIS2_PLACEMENT_3D('',#10285,#7734,#7735);
#6358=AXIS2_PLACEMENT_3D('',#10287,#7736,#7737);
#6359=AXIS2_PLACEMENT_3D('',#10289,#7738,#7739);
#6360=AXIS2_PLACEMENT_3D('',#10291,#7740,#7741);
#6361=AXIS2_PLACEMENT_3D('',#10293,#7742,#7743);
#6362=AXIS2_PLACEMENT_3D('',#10295,#7744,#7745);
#6363=AXIS2_PLACEMENT_3D('',#10297,#7746,#7747);
#6364=AXIS2_PLACEMENT_3D('',#10299,#7748,#7749);
#6365=AXIS2_PLACEMENT_3D('',#10301,#7750,#7751);
#6366=AXIS2_PLACEMENT_3D('',#10303,#7752,#7753);
#6367=AXIS2_PLACEMENT_3D('',#10305,#7754,#7755);
#6368=AXIS2_PLACEMENT_3D('',#10307,#7756,#7757);
#6369=AXIS2_PLACEMENT_3D('',#10309,#7758,#7759);
#6370=AXIS2_PLACEMENT_3D('',#10311,#7760,#7761);
#6371=AXIS2_PLACEMENT_3D('',#10313,#7762,#7763);
#6372=AXIS2_PLACEMENT_3D('',#10315,#7764,#7765);
#6373=AXIS2_PLACEMENT_3D('',#10317,#7766,#7767);
#6374=AXIS2_PLACEMENT_3D('',#10319,#7768,#7769);
#6375=AXIS2_PLACEMENT_3D('',#10321,#7770,#7771);
#6376=AXIS2_PLACEMENT_3D('',#10323,#7772,#7773);
#6377=AXIS2_PLACEMENT_3D('',#10325,#7774,#7775);
#6378=AXIS2_PLACEMENT_3D('',#10327,#7776,#7777);
#6379=AXIS2_PLACEMENT_3D('',#10329,#7778,#7779);
#6380=AXIS2_PLACEMENT_3D('',#10331,#7780,#7781);
#6381=AXIS2_PLACEMENT_3D('',#10333,#7782,#7783);
#6382=AXIS2_PLACEMENT_3D('',#10335,#7784,#7785);
#6383=AXIS2_PLACEMENT_3D('',#10337,#7786,#7787);
#6384=AXIS2_PLACEMENT_3D('',#10339,#7788,#7789);
#6385=AXIS2_PLACEMENT_3D('',#10341,#7790,#7791);
#6386=AXIS2_PLACEMENT_3D('',#10343,#7792,#7793);
#6387=AXIS2_PLACEMENT_3D('',#10345,#7794,#7795);
#6388=AXIS2_PLACEMENT_3D('',#10347,#7796,#7797);
#6389=AXIS2_PLACEMENT_3D('',#10349,#7798,#7799);
#6390=AXIS2_PLACEMENT_3D('',#10351,#7800,#7801);
#6391=AXIS2_PLACEMENT_3D('',#10352,#7802,#7803);
#6392=AXIS2_PLACEMENT_3D('',#10353,#7804,#7805);
#6393=AXIS2_PLACEMENT_3D('',#10355,#7807,#7808);
#6394=AXIS2_PLACEMENT_3D('',#10358,#7811,#7812);
#6395=AXIS2_PLACEMENT_3D('',#10360,#7814,#7815);
#6396=AXIS2_PLACEMENT_3D('',#10362,#7817,#7818);
#6397=AXIS2_PLACEMENT_3D('',#10364,#7820,#7821);
#6398=AXIS2_PLACEMENT_3D('',#10366,#7823,#7824);
#6399=AXIS2_PLACEMENT_3D('',#10368,#7826,#7827);
#6400=AXIS2_PLACEMENT_3D('',#10370,#7829,#7830);
#6401=AXIS2_PLACEMENT_3D('',#10372,#7832,#7833);
#6402=AXIS2_PLACEMENT_3D('',#10374,#7835,#7836);
#6403=AXIS2_PLACEMENT_3D('',#10376,#7838,#7839);
#6404=AXIS2_PLACEMENT_3D('',#10378,#7841,#7842);
#6405=AXIS2_PLACEMENT_3D('',#10380,#7844,#7845);
#6406=AXIS2_PLACEMENT_3D('',#10382,#7847,#7848);
#6407=AXIS2_PLACEMENT_3D('',#10384,#7850,#7851);
#6408=AXIS2_PLACEMENT_3D('',#10386,#7853,#7854);
#6409=AXIS2_PLACEMENT_3D('',#10388,#7856,#7857);
#6410=AXIS2_PLACEMENT_3D('',#10390,#7859,#7860);
#6411=AXIS2_PLACEMENT_3D('',#10392,#7862,#7863);
#6412=AXIS2_PLACEMENT_3D('',#10394,#7865,#7866);
#6413=AXIS2_PLACEMENT_3D('',#10396,#7868,#7869);
#6414=AXIS2_PLACEMENT_3D('',#10398,#7871,#7872);
#6415=AXIS2_PLACEMENT_3D('',#10400,#7874,#7875);
#6416=AXIS2_PLACEMENT_3D('',#10402,#7877,#7878);
#6417=AXIS2_PLACEMENT_3D('',#10404,#7880,#7881);
#6418=AXIS2_PLACEMENT_3D('',#10406,#7883,#7884);
#6419=AXIS2_PLACEMENT_3D('',#10408,#7886,#7887);
#6420=AXIS2_PLACEMENT_3D('',#10410,#7889,#7890);
#6421=AXIS2_PLACEMENT_3D('',#10412,#7892,#7893);
#6422=AXIS2_PLACEMENT_3D('',#10414,#7895,#7896);
#6423=AXIS2_PLACEMENT_3D('',#10416,#7898,#7899);
#6424=AXIS2_PLACEMENT_3D('',#10418,#7901,#7902);
#6425=AXIS2_PLACEMENT_3D('',#10420,#7904,#7905);
#6426=AXIS2_PLACEMENT_3D('',#10422,#7907,#7908);
#6427=AXIS2_PLACEMENT_3D('',#10424,#7910,#7911);
#6428=AXIS2_PLACEMENT_3D('',#10426,#7913,#7914);
#6429=AXIS2_PLACEMENT_3D('',#10428,#7916,#7917);
#6430=AXIS2_PLACEMENT_3D('',#10430,#7919,#7920);
#6431=AXIS2_PLACEMENT_3D('',#10432,#7922,#7923);
#6432=AXIS2_PLACEMENT_3D('',#10434,#7925,#7926);
#6433=AXIS2_PLACEMENT_3D('',#10436,#7928,#7929);
#6434=AXIS2_PLACEMENT_3D('',#10438,#7931,#7932);
#6435=AXIS2_PLACEMENT_3D('',#10440,#7934,#7935);
#6436=AXIS2_PLACEMENT_3D('',#10442,#7937,#7938);
#6437=AXIS2_PLACEMENT_3D('',#10444,#7940,#7941);
#6438=AXIS2_PLACEMENT_3D('',#10446,#7943,#7944);
#6439=AXIS2_PLACEMENT_3D('',#10448,#7946,#7947);
#6440=AXIS2_PLACEMENT_3D('',#10450,#7949,#7950);
#6441=AXIS2_PLACEMENT_3D('',#10452,#7952,#7953);
#6442=AXIS2_PLACEMENT_3D('',#10454,#7955,#7956);
#6443=AXIS2_PLACEMENT_3D('',#10456,#7958,#7959);
#6444=AXIS2_PLACEMENT_3D('',#10458,#7961,#7962);
#6445=AXIS2_PLACEMENT_3D('',#10460,#7964,#7965);
#6446=AXIS2_PLACEMENT_3D('',#10462,#7967,#7968);
#6447=AXIS2_PLACEMENT_3D('',#10464,#7970,#7971);
#6448=AXIS2_PLACEMENT_3D('',#10466,#7973,#7974);
#6449=AXIS2_PLACEMENT_3D('',#10468,#7976,#7977);
#6450=AXIS2_PLACEMENT_3D('',#10470,#7979,#7980);
#6451=AXIS2_PLACEMENT_3D('',#10472,#7982,#7983);
#6452=AXIS2_PLACEMENT_3D('',#10474,#7985,#7986);
#6453=AXIS2_PLACEMENT_3D('',#10476,#7988,#7989);
#6454=AXIS2_PLACEMENT_3D('',#10478,#7991,#7992);
#6455=AXIS2_PLACEMENT_3D('',#10480,#7994,#7995);
#6456=AXIS2_PLACEMENT_3D('',#10482,#7997,#7998);
#6457=AXIS2_PLACEMENT_3D('',#10484,#8000,#8001);
#6458=AXIS2_PLACEMENT_3D('',#10486,#8003,#8004);
#6459=AXIS2_PLACEMENT_3D('',#10488,#8006,#8007);
#6460=AXIS2_PLACEMENT_3D('',#10490,#8009,#8010);
#6461=AXIS2_PLACEMENT_3D('',#10492,#8012,#8013);
#6462=AXIS2_PLACEMENT_3D('',#10494,#8015,#8016);
#6463=AXIS2_PLACEMENT_3D('',#10496,#8018,#8019);
#6464=AXIS2_PLACEMENT_3D('',#10498,#8021,#8022);
#6465=AXIS2_PLACEMENT_3D('',#10500,#8024,#8025);
#6466=AXIS2_PLACEMENT_3D('',#10502,#8027,#8028);
#6467=AXIS2_PLACEMENT_3D('',#10504,#8030,#8031);
#6468=AXIS2_PLACEMENT_3D('',#10506,#8033,#8034);
#6469=AXIS2_PLACEMENT_3D('',#10508,#8036,#8037);
#6470=AXIS2_PLACEMENT_3D('',#10510,#8039,#8040);
#6471=AXIS2_PLACEMENT_3D('',#10512,#8042,#8043);
#6472=AXIS2_PLACEMENT_3D('',#10514,#8045,#8046);
#7417=DIRECTION('axis',(0.,0.,1.));
#7418=DIRECTION('refdir',(1.,0.,0.));
#7419=DIRECTION('center_axis',(-1.,0.,0.));
#7420=DIRECTION('ref_axis',(0.,0.,1.));
#7421=DIRECTION('',(0.,0.,1.));
#7422=DIRECTION('',(0.,1.,0.));
#7423=DIRECTION('',(0.,0.,-1.));
#7424=DIRECTION('',(0.,1.,0.));
#7425=DIRECTION('center_axis',(0.,0.,-1.));
#7426=DIRECTION('ref_axis',(-1.,0.,0.));
#7427=DIRECTION('',(-1.,0.,0.));
#7428=DIRECTION('',(0.,1.,0.));
#7429=DIRECTION('',(1.,0.,0.));
#7430=DIRECTION('center_axis',(0.,0.,1.));
#7431=DIRECTION('ref_axis',(1.,0.,0.));
#7432=DIRECTION('center_axis',(1.,0.,0.));
#7433=DIRECTION('ref_axis',(0.,0.,-1.));
#7434=DIRECTION('',(0.,0.,-1.));
#7435=DIRECTION('',(0.,-1.,0.));
#7436=DIRECTION('',(0.,0.,1.));
#7437=DIRECTION('center_axis',(0.,1.,0.));
#7438=DIRECTION('ref_axis',(1.,0.,0.));
#7439=DIRECTION('center_axis',(0.,1.,0.));
#7440=DIRECTION('ref_axis',(1.,0.,0.));
#7441=DIRECTION('center_axis',(0.,-1.,0.));
#7442=DIRECTION('ref_axis',(1.,0.,0.));
#7443=DIRECTION('center_axis',(0.,1.,0.));
#7444=DIRECTION('ref_axis',(-1.83697019872103E-16,0.,1.));
#7445=DIRECTION('center_axis',(0.,1.,0.));
#7446=DIRECTION('ref_axis',(1.,0.,0.));
#7447=DIRECTION('center_axis',(1.,0.,6.12323399573677E-17));
#7448=DIRECTION('ref_axis',(6.12323399573677E-17,0.,-1.));
#7449=DIRECTION('',(1.,0.,6.12323399573677E-17));
#7450=DIRECTION('center_axis',(1.,0.,6.12323399573677E-17));
#7451=DIRECTION('ref_axis',(6.12323399573677E-17,0.,-1.));
#7452=DIRECTION('',(1.,0.,6.12323399573677E-17));
#7453=DIRECTION('center_axis',(0.,-1.,0.));
#7454=DIRECTION('ref_axis',(1.,0.,0.));
#7455=DIRECTION('center_axis',(0.,-1.,0.));
#7456=DIRECTION('ref_axis',(1.,0.,0.));
#7457=DIRECTION('',(0.,1.,0.));
#7458=DIRECTION('',(0.,1.,0.));
#7459=DIRECTION('center_axis',(0.,1.,0.));
#7460=DIRECTION('ref_axis',(1.,0.,0.));
#7461=DIRECTION('center_axis',(0.,0.,1.));
#7462=DIRECTION('ref_axis',(1.,0.,0.));
#7463=DIRECTION('',(0.,0.,1.));
#7464=DIRECTION('center_axis',(0.,0.,1.));
#7465=DIRECTION('ref_axis',(1.,0.,0.));
#7466=DIRECTION('',(0.,0.,1.));
#7467=DIRECTION('center_axis',(0.,1.,0.));
#7468=DIRECTION('ref_axis',(1.,0.,0.));
#7469=DIRECTION('center_axis',(0.,1.,0.));
#7470=DIRECTION('ref_axis',(1.,0.,0.));
#7471=DIRECTION('center_axis',(0.,1.,0.));
#7472=DIRECTION('ref_axis',(1.,0.,0.));
#7473=DIRECTION('center_axis',(0.,1.,0.));
#7474=DIRECTION('ref_axis',(0.987688340595138,0.,0.156434465040231));
#7475=DIRECTION('center_axis',(0.,1.,0.));
#7476=DIRECTION('ref_axis',(1.,0.,0.));
#7477=DIRECTION('center_axis',(0.,1.,0.));
#7478=DIRECTION('ref_axis',(0.951056516295154,0.,0.309016994374948));
#7479=DIRECTION('center_axis',(0.,1.,0.));
#7480=DIRECTION('ref_axis',(1.,0.,0.));
#7481=DIRECTION('center_axis',(0.,1.,0.));
#7482=DIRECTION('ref_axis',(0.891006524188368,0.,0.453990499739547));
#7483=DIRECTION('center_axis',(0.,1.,0.));
#7484=DIRECTION('ref_axis',(1.,0.,0.));
#7485=DIRECTION('center_axis',(0.,1.,0.));
#7486=DIRECTION('ref_axis',(0.809016994374947,0.,0.587785252292473));
#7487=DIRECTION('center_axis',(0.,1.,0.));
#7488=DIRECTION('ref_axis',(1.,0.,0.));
#7489=DIRECTION('center_axis',(0.,1.,0.));
#7490=DIRECTION('ref_axis',(0.707106781186547,0.,0.707106781186548));
#7491=DIRECTION('center_axis',(0.,1.,0.));
#7492=DIRECTION('ref_axis',(1.,0.,0.));
#7493=DIRECTION('center_axis',(0.,1.,0.));
#7494=DIRECTION('ref_axis',(0.587785252292473,0.,0.809016994374948));
#7495=DIRECTION('center_axis',(0.,1.,0.));
#7496=DIRECTION('ref_axis',(1.,0.,0.));
#7497=DIRECTION('center_axis',(0.,1.,0.));
#7498=DIRECTION('ref_axis',(0.453990499739547,0.,0.891006524188368));
#7499=DIRECTION('center_axis',(0.,1.,0.));
#7500=DIRECTION('ref_axis',(1.,0.,0.));
#7501=DIRECTION('center_axis',(0.,1.,0.));
#7502=DIRECTION('ref_axis',(0.309016994374947,0.,0.951056516295154));
#7503=DIRECTION('center_axis',(0.,1.,0.));
#7504=DIRECTION('ref_axis',(1.,0.,0.));
#7505=DIRECTION('center_axis',(0.,1.,0.));
#7506=DIRECTION('ref_axis',(0.156434465040231,0.,0.987688340595138));
#7507=DIRECTION('center_axis',(0.,1.,0.));
#7508=DIRECTION('ref_axis',(1.,0.,0.));
#7509=DIRECTION('center_axis',(0.,1.,0.));
#7510=DIRECTION('ref_axis',(-1.83697019872103E-16,0.,1.));
#7511=DIRECTION('center_axis',(0.,1.,0.));
#7512=DIRECTION('ref_axis',(1.,0.,0.));
#7513=DIRECTION('center_axis',(0.,1.,0.));
#7514=DIRECTION('ref_axis',(-0.156434465040231,0.,0.987688340595138));
#7515=DIRECTION('center_axis',(0.,1.,0.));
#7516=DIRECTION('ref_axis',(1.,0.,0.));
#7517=DIRECTION('center_axis',(0.,1.,0.));
#7518=DIRECTION('ref_axis',(-0.309016994374948,0.,0.951056516295154));
#7519=DIRECTION('center_axis',(0.,1.,0.));
#7520=DIRECTION('ref_axis',(1.,0.,0.));
#7521=DIRECTION('center_axis',(0.,1.,0.));
#7522=DIRECTION('ref_axis',(-0.453990499739547,0.,0.891006524188368));
#7523=DIRECTION('center_axis',(0.,1.,0.));
#7524=DIRECTION('ref_axis',(1.,0.,0.));
#7525=DIRECTION('center_axis',(0.,1.,0.));
#7526=DIRECTION('ref_axis',(-0.587785252292473,0.,0.809016994374947));
#7527=DIRECTION('center_axis',(0.,1.,0.));
#7528=DIRECTION('ref_axis',(1.,0.,0.));
#7529=DIRECTION('center_axis',(0.,1.,0.));
#7530=DIRECTION('ref_axis',(-0.707106781186548,0.,0.707106781186547));
#7531=DIRECTION('center_axis',(0.,1.,0.));
#7532=DIRECTION('ref_axis',(1.,0.,0.));
#7533=DIRECTION('center_axis',(0.,1.,0.));
#7534=DIRECTION('ref_axis',(-0.809016994374947,0.,0.587785252292473));
#7535=DIRECTION('center_axis',(0.,1.,0.));
#7536=DIRECTION('ref_axis',(1.,0.,0.));
#7537=DIRECTION('center_axis',(0.,1.,0.));
#7538=DIRECTION('ref_axis',(-0.891006524188368,0.,0.453990499739547));
#7539=DIRECTION('center_axis',(0.,1.,0.));
#7540=DIRECTION('ref_axis',(1.,0.,0.));
#7541=DIRECTION('center_axis',(0.,1.,0.));
#7542=DIRECTION('ref_axis',(-0.951056516295154,0.,0.309016994374947));
#7543=DIRECTION('center_axis',(0.,1.,0.));
#7544=DIRECTION('ref_axis',(1.,0.,0.));
#7545=DIRECTION('center_axis',(0.,1.,0.));
#7546=DIRECTION('ref_axis',(-0.987688340595138,0.,0.156434465040231));
#7547=DIRECTION('center_axis',(0.,1.,0.));
#7548=DIRECTION('ref_axis',(1.,0.,0.));
#7549=DIRECTION('center_axis',(0.,1.,0.));
#7550=DIRECTION('ref_axis',(-1.,0.,-1.22464679914735E-16));
#7551=DIRECTION('center_axis',(0.,1.,0.));
#7552=DIRECTION('ref_axis',(1.,0.,0.));
#7553=DIRECTION('center_axis',(0.,1.,0.));
#7554=DIRECTION('ref_axis',(-0.987688340595138,0.,-0.156434465040231));
#7555=DIRECTION('center_axis',(0.,1.,0.));
#7556=DIRECTION('ref_axis',(1.,0.,0.));
#7557=DIRECTION('center_axis',(0.,1.,0.));
#7558=DIRECTION('ref_axis',(-0.951056516295154,0.,-0.309016994374948));
#7559=DIRECTION('center_axis',(0.,1.,0.));
#7560=DIRECTION('ref_axis',(1.,0.,0.));
#7561=DIRECTION('center_axis',(0.,1.,0.));
#7562=DIRECTION('ref_axis',(-0.891006524188368,0.,-0.453990499739547));
#7563=DIRECTION('center_axis',(0.,1.,0.));
#7564=DIRECTION('ref_axis',(1.,0.,0.));
#7565=DIRECTION('center_axis',(0.,1.,0.));
#7566=DIRECTION('ref_axis',(-0.809016994374947,0.,-0.587785252292473));
#7567=DIRECTION('center_axis',(0.,1.,0.));
#7568=DIRECTION('ref_axis',(1.,0.,0.));
#7569=DIRECTION('center_axis',(0.,1.,0.));
#7570=DIRECTION('ref_axis',(-0.707106781186547,0.,-0.707106781186548));
#7571=DIRECTION('center_axis',(0.,1.,0.));
#7572=DIRECTION('ref_axis',(1.,0.,0.));
#7573=DIRECTION('center_axis',(0.,1.,0.));
#7574=DIRECTION('ref_axis',(-0.587785252292473,0.,-0.809016994374947));
#7575=DIRECTION('center_axis',(0.,1.,0.));
#7576=DIRECTION('ref_axis',(1.,0.,0.));
#7577=DIRECTION('center_axis',(0.,1.,0.));
#7578=DIRECTION('ref_axis',(-0.453990499739547,0.,-0.891006524188368));
#7579=DIRECTION('center_axis',(0.,1.,0.));
#7580=DIRECTION('ref_axis',(1.,0.,0.));
#7581=DIRECTION('center_axis',(0.,1.,0.));
#7582=DIRECTION('ref_axis',(-0.309016994374947,0.,-0.951056516295154));
#7583=DIRECTION('center_axis',(0.,1.,0.));
#7584=DIRECTION('ref_axis',(1.,0.,0.));
#7585=DIRECTION('center_axis',(0.,1.,0.));
#7586=DIRECTION('ref_axis',(-0.156434465040231,0.,-0.987688340595138));
#7587=DIRECTION('center_axis',(0.,1.,0.));
#7588=DIRECTION('ref_axis',(1.,0.,0.));
#7589=DIRECTION('center_axis',(0.,1.,0.));
#7590=DIRECTION('ref_axis',(6.12323399573677E-17,0.,-1.));
#7591=DIRECTION('center_axis',(0.,1.,0.));
#7592=DIRECTION('ref_axis',(1.,0.,0.));
#7593=DIRECTION('center_axis',(0.,1.,0.));
#7594=DIRECTION('ref_axis',(0.156434465040231,0.,-0.987688340595138));
#7595=DIRECTION('center_axis',(0.,1.,0.));
#7596=DIRECTION('ref_axis',(1.,0.,0.));
#7597=DIRECTION('center_axis',(0.,1.,0.));
#7598=DIRECTION('ref_axis',(0.309016994374948,0.,-0.951056516295154));
#7599=DIRECTION('center_axis',(0.,1.,0.));
#7600=DIRECTION('ref_axis',(1.,0.,0.));
#7601=DIRECTION('center_axis',(0.,1.,0.));
#7602=DIRECTION('ref_axis',(0.453990499739547,0.,-0.891006524188368));
#7603=DIRECTION('center_axis',(0.,1.,0.));
#7604=DIRECTION('ref_axis',(1.,0.,0.));
#7605=DIRECTION('center_axis',(0.,1.,0.));
#7606=DIRECTION('ref_axis',(0.587785252292473,0.,-0.809016994374947));
#7607=DIRECTION('center_axis',(0.,1.,0.));
#7608=DIRECTION('ref_axis',(1.,0.,0.));
#7609=DIRECTION('center_axis',(0.,1.,0.));
#7610=DIRECTION('ref_axis',(0.707106781186548,0.,-0.707106781186547));
#7611=DIRECTION('center_axis',(0.,1.,0.));
#7612=DIRECTION('ref_axis',(1.,0.,0.));
#7613=DIRECTION('center_axis',(0.,1.,0.));
#7614=DIRECTION('ref_axis',(0.809016994374947,0.,-0.587785252292473));
#7615=DIRECTION('center_axis',(0.,1.,0.));
#7616=DIRECTION('ref_axis',(1.,0.,0.));
#7617=DIRECTION('center_axis',(0.,1.,0.));
#7618=DIRECTION('ref_axis',(0.891006524188368,0.,-0.453990499739547));
#7619=DIRECTION('center_axis',(0.,1.,0.));
#7620=DIRECTION('ref_axis',(1.,0.,0.));
#7621=DIRECTION('center_axis',(0.,1.,0.));
#7622=DIRECTION('ref_axis',(0.951056516295154,0.,-0.309016994374947));
#7623=DIRECTION('center_axis',(0.,1.,0.));
#7624=DIRECTION('ref_axis',(1.,0.,0.));
#7625=DIRECTION('center_axis',(0.,1.,0.));
#7626=DIRECTION('ref_axis',(0.987688340595138,0.,-0.156434465040231));
#7627=DIRECTION('center_axis',(0.,1.,0.));
#7628=DIRECTION('ref_axis',(1.,0.,0.));
#7629=DIRECTION('center_axis',(0.,1.,0.));
#7630=DIRECTION('ref_axis',(1.,0.,0.));
#7631=DIRECTION('center_axis',(0.,1.,0.));
#7632=DIRECTION('ref_axis',(1.,0.,0.));
#7633=DIRECTION('center_axis',(0.,-1.,0.));
#7634=DIRECTION('ref_axis',(1.,0.,0.));
#7635=DIRECTION('center_axis',(0.,-1.,0.));
#7636=DIRECTION('ref_axis',(1.,0.,0.));
#7637=DIRECTION('',(0.,1.,0.));
#7638=DIRECTION('center_axis',(0.,1.,0.));
#7639=DIRECTION('ref_axis',(1.,0.,0.));
#7640=DIRECTION('center_axis',(0.,1.,0.));
#7641=DIRECTION('ref_axis',(1.,0.,0.));
#7642=DIRECTION('center_axis',(0.,1.,0.));
#7643=DIRECTION('ref_axis',(1.,0.,0.));
#7644=DIRECTION('center_axis',(0.,-1.,0.));
#7645=DIRECTION('ref_axis',(0.987688340595138,0.,0.156434465040231));
#7646=DIRECTION('center_axis',(0.,1.,0.));
#7647=DIRECTION('ref_axis',(1.,0.,0.));
#7648=DIRECTION('center_axis',(0.,-1.,0.));
#7649=DIRECTION('ref_axis',(1.,0.,0.));
#7650=DIRECTION('center_axis',(0.,1.,0.));
#7651=DIRECTION('ref_axis',(1.,0.,0.));
#7652=DIRECTION('center_axis',(0.,-1.,0.));
#7653=DIRECTION('ref_axis',(0.987688340595138,0.,-0.156434465040231));
#7654=DIRECTION('center_axis',(0.,1.,0.));
#7655=DIRECTION('ref_axis',(1.,0.,0.));
#7656=DIRECTION('center_axis',(0.,-1.,0.));
#7657=DIRECTION('ref_axis',(0.951056516295154,0.,-0.309016994374947));
#7658=DIRECTION('center_axis',(0.,1.,0.));
#7659=DIRECTION('ref_axis',(1.,0.,0.));
#7660=DIRECTION('center_axis',(0.,-1.,0.));
#7661=DIRECTION('ref_axis',(0.891006524188368,0.,-0.453990499739547));
#7662=DIRECTION('center_axis',(0.,1.,0.));
#7663=DIRECTION('ref_axis',(1.,0.,0.));
#7664=DIRECTION('center_axis',(0.,-1.,0.));
#7665=DIRECTION('ref_axis',(0.809016994374947,0.,-0.587785252292473));
#7666=DIRECTION('center_axis',(0.,1.,0.));
#7667=DIRECTION('ref_axis',(1.,0.,0.));
#7668=DIRECTION('center_axis',(0.,-1.,0.));
#7669=DIRECTION('ref_axis',(0.707106781186548,0.,-0.707106781186547));
#7670=DIRECTION('center_axis',(0.,1.,0.));
#7671=DIRECTION('ref_axis',(1.,0.,0.));
#7672=DIRECTION('center_axis',(0.,-1.,0.));
#7673=DIRECTION('ref_axis',(0.587785252292473,0.,-0.809016994374947));
#7674=DIRECTION('center_axis',(0.,1.,0.));
#7675=DIRECTION('ref_axis',(1.,0.,0.));
#7676=DIRECTION('center_axis',(0.,-1.,0.));
#7677=DIRECTION('ref_axis',(0.453990499739547,0.,-0.891006524188368));
#7678=DIRECTION('center_axis',(0.,1.,0.));
#7679=DIRECTION('ref_axis',(1.,0.,0.));
#7680=DIRECTION('center_axis',(0.,-1.,0.));
#7681=DIRECTION('ref_axis',(0.309016994374948,0.,-0.951056516295154));
#7682=DIRECTION('center_axis',(0.,1.,0.));
#7683=DIRECTION('ref_axis',(1.,0.,0.));
#7684=DIRECTION('center_axis',(0.,-1.,0.));
#7685=DIRECTION('ref_axis',(0.156434465040231,0.,-0.987688340595138));
#7686=DIRECTION('center_axis',(0.,1.,0.));
#7687=DIRECTION('ref_axis',(1.,0.,0.));
#7688=DIRECTION('center_axis',(0.,-1.,0.));
#7689=DIRECTION('ref_axis',(6.12323399573677E-17,0.,-1.));
#7690=DIRECTION('center_axis',(0.,1.,0.));
#7691=DIRECTION('ref_axis',(1.,0.,0.));
#7692=DIRECTION('center_axis',(0.,-1.,0.));
#7693=DIRECTION('ref_axis',(-0.156434465040231,0.,-0.987688340595138));
#7694=DIRECTION('center_axis',(0.,1.,0.));
#7695=DIRECTION('ref_axis',(1.,0.,0.));
#7696=DIRECTION('center_axis',(0.,-1.,0.));
#7697=DIRECTION('ref_axis',(-0.309016994374947,0.,-0.951056516295154));
#7698=DIRECTION('center_axis',(0.,1.,0.));
#7699=DIRECTION('ref_axis',(1.,0.,0.));
#7700=DIRECTION('center_axis',(0.,-1.,0.));
#7701=DIRECTION('ref_axis',(-0.453990499739547,0.,-0.891006524188368));
#7702=DIRECTION('center_axis',(0.,1.,0.));
#7703=DIRECTION('ref_axis',(1.,0.,0.));
#7704=DIRECTION('center_axis',(0.,-1.,0.));
#7705=DIRECTION('ref_axis',(-0.587785252292473,0.,-0.809016994374947));
#7706=DIRECTION('center_axis',(0.,1.,0.));
#7707=DIRECTION('ref_axis',(1.,0.,0.));
#7708=DIRECTION('center_axis',(0.,-1.,0.));
#7709=DIRECTION('ref_axis',(-0.707106781186547,0.,-0.707106781186548));
#7710=DIRECTION('center_axis',(0.,1.,0.));
#7711=DIRECTION('ref_axis',(1.,0.,0.));
#7712=DIRECTION('center_axis',(0.,-1.,0.));
#7713=DIRECTION('ref_axis',(-0.809016994374947,0.,-0.587785252292473));
#7714=DIRECTION('center_axis',(0.,1.,0.));
#7715=DIRECTION('ref_axis',(1.,0.,0.));
#7716=DIRECTION('center_axis',(0.,-1.,0.));
#7717=DIRECTION('ref_axis',(-0.891006524188368,0.,-0.453990499739547));
#7718=DIRECTION('center_axis',(0.,1.,0.));
#7719=DIRECTION('ref_axis',(1.,0.,0.));
#7720=DIRECTION('center_axis',(0.,-1.,0.));
#7721=DIRECTION('ref_axis',(-0.951056516295154,0.,-0.309016994374948));
#7722=DIRECTION('center_axis',(0.,1.,0.));
#7723=DIRECTION('ref_axis',(1.,0.,0.));
#7724=DIRECTION('center_axis',(0.,-1.,0.));
#7725=DIRECTION('ref_axis',(-0.987688340595138,0.,-0.156434465040231));
#7726=DIRECTION('center_axis',(0.,1.,0.));
#7727=DIRECTION('ref_axis',(1.,0.,0.));
#7728=DIRECTION('center_axis',(0.,-1.,0.));
#7729=DIRECTION('ref_axis',(-1.,0.,-1.22464679914735E-16));
#7730=DIRECTION('center_axis',(0.,1.,0.));
#7731=DIRECTION('ref_axis',(1.,0.,0.));
#7732=DIRECTION('center_axis',(0.,-1.,0.));
#7733=DIRECTION('ref_axis',(-0.987688340595138,0.,0.156434465040231));
#7734=DIRECTION('center_axis',(0.,1.,0.));
#7735=DIRECTION('ref_axis',(1.,0.,0.));
#7736=DIRECTION('center_axis',(0.,-1.,0.));
#7737=DIRECTION('ref_axis',(-0.951056516295154,0.,0.309016994374947));
#7738=DIRECTION('center_axis',(0.,1.,0.));
#7739=DIRECTION('ref_axis',(1.,0.,0.));
#7740=DIRECTION('center_axis',(0.,-1.,0.));
#7741=DIRECTION('ref_axis',(-0.891006524188368,0.,0.453990499739547));
#7742=DIRECTION('center_axis',(0.,1.,0.));
#7743=DIRECTION('ref_axis',(1.,0.,0.));
#7744=DIRECTION('center_axis',(0.,-1.,0.));
#7745=DIRECTION('ref_axis',(-0.809016994374947,0.,0.587785252292473));
#7746=DIRECTION('center_axis',(0.,1.,0.));
#7747=DIRECTION('ref_axis',(1.,0.,0.));
#7748=DIRECTION('center_axis',(0.,-1.,0.));
#7749=DIRECTION('ref_axis',(-0.707106781186548,0.,0.707106781186547));
#7750=DIRECTION('center_axis',(0.,1.,0.));
#7751=DIRECTION('ref_axis',(1.,0.,0.));
#7752=DIRECTION('center_axis',(0.,-1.,0.));
#7753=DIRECTION('ref_axis',(-0.587785252292473,0.,0.809016994374947));
#7754=DIRECTION('center_axis',(0.,1.,0.));
#7755=DIRECTION('ref_axis',(1.,0.,0.));
#7756=DIRECTION('center_axis',(0.,-1.,0.));
#7757=DIRECTION('ref_axis',(-0.453990499739547,0.,0.891006524188368));
#7758=DIRECTION('center_axis',(0.,1.,0.));
#7759=DIRECTION('ref_axis',(1.,0.,0.));
#7760=DIRECTION('center_axis',(0.,-1.,0.));
#7761=DIRECTION('ref_axis',(-0.309016994374948,0.,0.951056516295154));
#7762=DIRECTION('center_axis',(0.,1.,0.));
#7763=DIRECTION('ref_axis',(1.,0.,0.));
#7764=DIRECTION('center_axis',(0.,-1.,0.));
#7765=DIRECTION('ref_axis',(-0.156434465040231,0.,0.987688340595138));
#7766=DIRECTION('center_axis',(0.,1.,0.));
#7767=DIRECTION('ref_axis',(1.,0.,0.));
#7768=DIRECTION('center_axis',(0.,-1.,0.));
#7769=DIRECTION('ref_axis',(-1.83697019872103E-16,0.,1.));
#7770=DIRECTION('center_axis',(0.,1.,0.));
#7771=DIRECTION('ref_axis',(1.,0.,0.));
#7772=DIRECTION('center_axis',(0.,-1.,0.));
#7773=DIRECTION('ref_axis',(0.156434465040231,0.,0.987688340595138));
#7774=DIRECTION('center_axis',(0.,1.,0.));
#7775=DIRECTION('ref_axis',(1.,0.,0.));
#7776=DIRECTION('center_axis',(0.,-1.,0.));
#7777=DIRECTION('ref_axis',(0.309016994374947,0.,0.951056516295154));
#7778=DIRECTION('center_axis',(0.,1.,0.));
#7779=DIRECTION('ref_axis',(1.,0.,0.));
#7780=DIRECTION('center_axis',(0.,-1.,0.));
#7781=DIRECTION('ref_axis',(0.453990499739547,0.,0.891006524188368));
#7782=DIRECTION('center_axis',(0.,1.,0.));
#7783=DIRECTION('ref_axis',(1.,0.,0.));
#7784=DIRECTION('center_axis',(0.,-1.,0.));
#7785=DIRECTION('ref_axis',(0.587785252292473,0.,0.809016994374948));
#7786=DIRECTION('center_axis',(0.,1.,0.));
#7787=DIRECTION('ref_axis',(1.,0.,0.));
#7788=DIRECTION('center_axis',(0.,-1.,0.));
#7789=DIRECTION('ref_axis',(0.707106781186547,0.,0.707106781186548));
#7790=DIRECTION('center_axis',(0.,1.,0.));
#7791=DIRECTION('ref_axis',(1.,0.,0.));
#7792=DIRECTION('center_axis',(0.,-1.,0.));
#7793=DIRECTION('ref_axis',(0.809016994374947,0.,0.587785252292473));
#7794=DIRECTION('center_axis',(0.,1.,0.));
#7795=DIRECTION('ref_axis',(1.,0.,0.));
#7796=DIRECTION('center_axis',(0.,-1.,0.));
#7797=DIRECTION('ref_axis',(0.891006524188368,0.,0.453990499739547));
#7798=DIRECTION('center_axis',(0.,1.,0.));
#7799=DIRECTION('ref_axis',(1.,0.,0.));
#7800=DIRECTION('center_axis',(0.,-1.,0.));
#7801=DIRECTION('ref_axis',(0.951056516295154,0.,0.309016994374948));
#7802=DIRECTION('center_axis',(0.,1.,0.));
#7803=DIRECTION('ref_axis',(1.,0.,0.));
#7804=DIRECTION('center_axis',(0.,1.,0.));
#7805=DIRECTION('ref_axis',(1.,0.,0.));
#7806=DIRECTION('',(0.,-1.,0.));
#7807=DIRECTION('center_axis',(0.,1.,0.));
#7808=DIRECTION('ref_axis',(-0.987688340595137,0.,-0.156434465040233));
#7809=DIRECTION('',(0.,-1.,0.));
#7810=DIRECTION('',(0.,1.,0.));
#7811=DIRECTION('center_axis',(0.,1.,0.));
#7812=DIRECTION('ref_axis',(1.,0.,0.));
#7813=DIRECTION('',(0.,-1.,0.));
#7814=DIRECTION('center_axis',(0.,1.,0.));
#7815=DIRECTION('ref_axis',(-0.951056516295153,0.,-0.309016994374949));
#7816=DIRECTION('',(0.,1.,0.));
#7817=DIRECTION('center_axis',(0.,1.,0.));
#7818=DIRECTION('ref_axis',(1.,0.,0.));
#7819=DIRECTION('',(0.,-1.,0.));
#7820=DIRECTION('center_axis',(0.,1.,0.));
#7821=DIRECTION('ref_axis',(-0.891006524188368,0.,-0.453990499739547));
#7822=DIRECTION('',(0.,1.,0.));
#7823=DIRECTION('center_axis',(0.,1.,0.));
#7824=DIRECTION('ref_axis',(1.,0.,0.));
#7825=DIRECTION('',(0.,-1.,0.));
#7826=DIRECTION('center_axis',(0.,1.,0.));
#7827=DIRECTION('ref_axis',(-0.809016994374948,0.,-0.587785252292473));
#7828=DIRECTION('',(0.,1.,0.));
#7829=DIRECTION('center_axis',(0.,1.,0.));
#7830=DIRECTION('ref_axis',(1.,0.,0.));
#7831=DIRECTION('',(0.,-1.,0.));
#7832=DIRECTION('center_axis',(0.,1.,0.));
#7833=DIRECTION('ref_axis',(-0.707106781186547,0.,-0.707106781186548));
#7834=DIRECTION('',(0.,1.,0.));
#7835=DIRECTION('center_axis',(0.,1.,0.));
#7836=DIRECTION('ref_axis',(1.,0.,0.));
#7837=DIRECTION('',(0.,-1.,0.));
#7838=DIRECTION('center_axis',(0.,1.,0.));
#7839=DIRECTION('ref_axis',(-0.587785252292474,0.,-0.809016994374947));
#7840=DIRECTION('',(0.,1.,0.));
#7841=DIRECTION('center_axis',(0.,1.,0.));
#7842=DIRECTION('ref_axis',(1.,0.,0.));
#7843=DIRECTION('',(0.,-1.,0.));
#7844=DIRECTION('center_axis',(0.,1.,0.));
#7845=DIRECTION('ref_axis',(-0.453990499739547,0.,-0.891006524188368));
#7846=DIRECTION('',(0.,1.,0.));
#7847=DIRECTION('center_axis',(0.,1.,0.));
#7848=DIRECTION('ref_axis',(1.,0.,0.));
#7849=DIRECTION('',(0.,-1.,0.));
#7850=DIRECTION('center_axis',(0.,1.,0.));
#7851=DIRECTION('ref_axis',(-0.309016994374948,0.,-0.951056516295153));
#7852=DIRECTION('',(0.,1.,0.));
#7853=DIRECTION('center_axis',(0.,1.,0.));
#7854=DIRECTION('ref_axis',(1.,0.,0.));
#7855=DIRECTION('',(0.,-1.,0.));
#7856=DIRECTION('center_axis',(0.,1.,0.));
#7857=DIRECTION('ref_axis',(-0.156434465040232,0.,-0.987688340595138));
#7858=DIRECTION('',(0.,1.,0.));
#7859=DIRECTION('center_axis',(0.,1.,0.));
#7860=DIRECTION('ref_axis',(1.,0.,0.));
#7861=DIRECTION('',(0.,-1.,0.));
#7862=DIRECTION('center_axis',(0.,1.,0.));
#7863=DIRECTION('ref_axis',(3.06161699786838E-16,0.,-1.));
#7864=DIRECTION('',(0.,1.,0.));
#7865=DIRECTION('center_axis',(0.,1.,0.));
#7866=DIRECTION('ref_axis',(1.,0.,0.));
#7867=DIRECTION('',(0.,-1.,0.));
#7868=DIRECTION('center_axis',(0.,1.,0.));
#7869=DIRECTION('ref_axis',(0.156434465040233,0.,-0.987688340595138));
#7870=DIRECTION('',(0.,1.,0.));
#7871=DIRECTION('center_axis',(0.,1.,0.));
#7872=DIRECTION('ref_axis',(1.,0.,0.));
#7873=DIRECTION('',(0.,-1.,0.));
#7874=DIRECTION('center_axis',(0.,1.,0.));
#7875=DIRECTION('ref_axis',(0.309016994374946,0.,-0.951056516295154));
#7876=DIRECTION('',(0.,1.,0.));
#7877=DIRECTION('center_axis',(0.,1.,0.));
#7878=DIRECTION('ref_axis',(1.,0.,0.));
#7879=DIRECTION('',(0.,-1.,0.));
#7880=DIRECTION('center_axis',(0.,1.,0.));
#7881=DIRECTION('ref_axis',(0.453990499739547,0.,-0.891006524188368));
#7882=DIRECTION('',(0.,1.,0.));
#7883=DIRECTION('center_axis',(0.,1.,0.));
#7884=DIRECTION('ref_axis',(1.,0.,0.));
#7885=DIRECTION('',(0.,-1.,0.));
#7886=DIRECTION('center_axis',(0.,1.,0.));
#7887=DIRECTION('ref_axis',(0.587785252292473,0.,-0.809016994374947));
#7888=DIRECTION('',(0.,1.,0.));
#7889=DIRECTION('center_axis',(0.,1.,0.));
#7890=DIRECTION('ref_axis',(1.,0.,0.));
#7891=DIRECTION('',(0.,-1.,0.));
#7892=DIRECTION('center_axis',(0.,1.,0.));
#7893=DIRECTION('ref_axis',(0.707106781186548,0.,-0.707106781186547));
#7894=DIRECTION('',(0.,1.,0.));
#7895=DIRECTION('center_axis',(0.,1.,0.));
#7896=DIRECTION('ref_axis',(1.,0.,0.));
#7897=DIRECTION('',(0.,-1.,0.));
#7898=DIRECTION('center_axis',(0.,1.,0.));
#7899=DIRECTION('ref_axis',(0.809016994374946,0.,-0.587785252292475));
#7900=DIRECTION('',(0.,1.,0.));
#7901=DIRECTION('center_axis',(0.,1.,0.));
#7902=DIRECTION('ref_axis',(1.,0.,0.));
#7903=DIRECTION('',(0.,-1.,0.));
#7904=DIRECTION('center_axis',(0.,1.,0.));
#7905=DIRECTION('ref_axis',(0.891006524188368,0.,-0.453990499739547));
#7906=DIRECTION('',(0.,1.,0.));
#7907=DIRECTION('center_axis',(0.,1.,0.));
#7908=DIRECTION('ref_axis',(1.,0.,0.));
#7909=DIRECTION('',(0.,-1.,0.));
#7910=DIRECTION('center_axis',(0.,1.,0.));
#7911=DIRECTION('ref_axis',(0.951056516295154,0.,-0.309016994374946));
#7912=DIRECTION('',(0.,1.,0.));
#7913=DIRECTION('center_axis',(0.,1.,0.));
#7914=DIRECTION('ref_axis',(1.,0.,0.));
#7915=DIRECTION('',(0.,-1.,0.));
#7916=DIRECTION('center_axis',(0.,1.,0.));
#7917=DIRECTION('ref_axis',(0.987688340595138,0.,-0.156434465040232));
#7918=DIRECTION('',(0.,1.,0.));
#7919=DIRECTION('center_axis',(0.,1.,0.));
#7920=DIRECTION('ref_axis',(1.,0.,0.));
#7921=DIRECTION('',(0.,-1.,0.));
#7922=DIRECTION('center_axis',(0.,1.,0.));
#7923=DIRECTION('ref_axis',(1.,0.,2.44929359829471E-16));
#7924=DIRECTION('',(0.,1.,0.));
#7925=DIRECTION('center_axis',(0.,1.,0.));
#7926=DIRECTION('ref_axis',(1.,0.,0.));
#7927=DIRECTION('',(0.,-1.,0.));
#7928=DIRECTION('center_axis',(0.,1.,0.));
#7929=DIRECTION('ref_axis',(0.987688340595137,0.,0.156434465040232));
#7930=DIRECTION('',(0.,1.,0.));
#7931=DIRECTION('center_axis',(0.,1.,0.));
#7932=DIRECTION('ref_axis',(1.,0.,0.));
#7933=DIRECTION('',(0.,-1.,0.));
#7934=DIRECTION('center_axis',(0.,1.,0.));
#7935=DIRECTION('ref_axis',(0.951056516295154,0.,0.309016994374946));
#7936=DIRECTION('',(0.,1.,0.));
#7937=DIRECTION('center_axis',(0.,1.,0.));
#7938=DIRECTION('ref_axis',(1.,0.,0.));
#7939=DIRECTION('',(0.,-1.,0.));
#7940=DIRECTION('center_axis',(0.,1.,0.));
#7941=DIRECTION('ref_axis',(0.891006524188368,0.,0.453990499739547));
#7942=DIRECTION('',(0.,1.,0.));
#7943=DIRECTION('center_axis',(0.,1.,0.));
#7944=DIRECTION('ref_axis',(1.,0.,0.));
#7945=DIRECTION('',(0.,-1.,0.));
#7946=DIRECTION('center_axis',(0.,1.,0.));
#7947=DIRECTION('ref_axis',(0.809016994374947,0.,0.587785252292473));
#7948=DIRECTION('',(0.,1.,0.));
#7949=DIRECTION('center_axis',(0.,1.,0.));
#7950=DIRECTION('ref_axis',(1.,0.,0.));
#7951=DIRECTION('',(0.,-1.,0.));
#7952=DIRECTION('center_axis',(0.,1.,0.));
#7953=DIRECTION('ref_axis',(0.707106781186547,0.,0.707106781186548));
#7954=DIRECTION('',(0.,1.,0.));
#7955=DIRECTION('center_axis',(0.,1.,0.));
#7956=DIRECTION('ref_axis',(1.,0.,0.));
#7957=DIRECTION('',(0.,-1.,0.));
#7958=DIRECTION('center_axis',(0.,1.,0.));
#7959=DIRECTION('ref_axis',(0.587785252292475,0.,0.809016994374946));
#7960=DIRECTION('',(0.,1.,0.));
#7961=DIRECTION('center_axis',(0.,1.,0.));
#7962=DIRECTION('ref_axis',(1.,0.,0.));
#7963=DIRECTION('',(0.,-1.,0.));
#7964=DIRECTION('center_axis',(0.,1.,0.));
#7965=DIRECTION('ref_axis',(0.453990499739547,0.,0.891006524188368));
#7966=DIRECTION('',(0.,1.,0.));
#7967=DIRECTION('center_axis',(0.,1.,0.));
#7968=DIRECTION('ref_axis',(1.,0.,0.));
#7969=DIRECTION('',(0.,-1.,0.));
#7970=DIRECTION('center_axis',(0.,1.,0.));
#7971=DIRECTION('ref_axis',(0.309016994374946,0.,0.951056516295154));
#7972=DIRECTION('',(0.,1.,0.));
#7973=DIRECTION('center_axis',(0.,1.,0.));
#7974=DIRECTION('ref_axis',(1.,0.,0.));
#7975=DIRECTION('',(0.,-1.,0.));
#7976=DIRECTION('center_axis',(0.,1.,0.));
#7977=DIRECTION('ref_axis',(0.156434465040232,0.,0.987688340595138));
#7978=DIRECTION('',(0.,1.,0.));
#7979=DIRECTION('center_axis',(0.,1.,0.));
#7980=DIRECTION('ref_axis',(1.,0.,0.));
#7981=DIRECTION('',(0.,-1.,0.));
#7982=DIRECTION('center_axis',(0.,1.,0.));
#7983=DIRECTION('ref_axis',(-1.83697019872103E-16,0.,1.));
#7984=DIRECTION('',(0.,1.,0.));
#7985=DIRECTION('center_axis',(0.,1.,0.));
#7986=DIRECTION('ref_axis',(1.,0.,0.));
#7987=DIRECTION('',(0.,-1.,0.));
#7988=DIRECTION('center_axis',(0.,1.,0.));
#7989=DIRECTION('ref_axis',(-0.156434465040232,0.,0.987688340595138));
#7990=DIRECTION('',(0.,1.,0.));
#7991=DIRECTION('center_axis',(0.,1.,0.));
#7992=DIRECTION('ref_axis',(1.,0.,0.));
#7993=DIRECTION('',(0.,-1.,0.));
#7994=DIRECTION('center_axis',(0.,1.,0.));
#7995=DIRECTION('ref_axis',(-0.309016994374946,0.,0.951056516295154));
#7996=DIRECTION('',(0.,1.,0.));
#7997=DIRECTION('center_axis',(0.,1.,0.));
#7998=DIRECTION('ref_axis',(1.,0.,0.));
#7999=DIRECTION('',(0.,-1.,0.));
#8000=DIRECTION('center_axis',(0.,1.,0.));
#8001=DIRECTION('ref_axis',(-0.453990499739549,0.,0.891006524188367));
#8002=DIRECTION('',(0.,1.,0.));
#8003=DIRECTION('center_axis',(0.,1.,0.));
#8004=DIRECTION('ref_axis',(1.,0.,0.));
#8005=DIRECTION('',(0.,-1.,0.));
#8006=DIRECTION('center_axis',(0.,1.,0.));
#8007=DIRECTION('ref_axis',(-0.587785252292474,0.,0.809016994374947));
#8008=DIRECTION('',(0.,1.,0.));
#8009=DIRECTION('center_axis',(0.,1.,0.));
#8010=DIRECTION('ref_axis',(1.,0.,0.));
#8011=DIRECTION('',(0.,-1.,0.));
#8012=DIRECTION('center_axis',(0.,1.,0.));
#8013=DIRECTION('ref_axis',(-0.707106781186548,0.,0.707106781186547));
#8014=DIRECTION('',(0.,1.,0.));
#8015=DIRECTION('center_axis',(0.,1.,0.));
#8016=DIRECTION('ref_axis',(1.,0.,0.));
#8017=DIRECTION('',(0.,-1.,0.));
#8018=DIRECTION('center_axis',(0.,1.,0.));
#8019=DIRECTION('ref_axis',(-0.809016994374947,0.,0.587785252292474));
#8020=DIRECTION('',(0.,1.,0.));
#8021=DIRECTION('center_axis',(0.,1.,0.));
#8022=DIRECTION('ref_axis',(1.,0.,0.));
#8023=DIRECTION('',(0.,-1.,0.));
#8024=DIRECTION('center_axis',(0.,1.,0.));
#8025=DIRECTION('ref_axis',(-0.891006524188368,0.,0.453990499739547));
#8026=DIRECTION('',(0.,1.,0.));
#8027=DIRECTION('center_axis',(0.,1.,0.));
#8028=DIRECTION('ref_axis',(1.,0.,0.));
#8029=DIRECTION('',(0.,-1.,0.));
#8030=DIRECTION('center_axis',(0.,1.,0.));
#8031=DIRECTION('ref_axis',(-0.951056516295154,0.,0.309016994374948));
#8032=DIRECTION('',(0.,1.,0.));
#8033=DIRECTION('center_axis',(0.,1.,0.));
#8034=DIRECTION('ref_axis',(1.,0.,0.));
#8035=DIRECTION('',(0.,-1.,0.));
#8036=DIRECTION('center_axis',(0.,1.,0.));
#8037=DIRECTION('ref_axis',(-0.987688340595137,0.,0.156434465040233));
#8038=DIRECTION('',(0.,1.,0.));
#8039=DIRECTION('center_axis',(0.,1.,0.));
#8040=DIRECTION('ref_axis',(1.,0.,0.));
#8041=DIRECTION('',(0.,1.,0.));
#8042=DIRECTION('center_axis',(0.,1.,0.));
#8043=DIRECTION('ref_axis',(-1.,0.,-1.22464679914735E-16));
#8044=DIRECTION('',(0.,-1.,0.));
#8045=DIRECTION('center_axis',(0.,1.,0.));
#8046=DIRECTION('ref_axis',(1.,0.,0.));
#9698=CARTESIAN_POINT('',(0.,0.,0.));
#9699=CARTESIAN_POINT('Origin',(-0.2,-1.,-0.78));
#9700=CARTESIAN_POINT('',(-0.2,-0.9,-0.78));
#9701=CARTESIAN_POINT('',(-0.2,-0.9,-0.565685424949238));
#9702=CARTESIAN_POINT('',(-0.2,-0.9,-0.39));
#9703=CARTESIAN_POINT('',(-0.2,0.85,-0.78));
#9704=CARTESIAN_POINT('',(-0.2,-1.,-0.78));
#9705=CARTESIAN_POINT('',(-0.2,0.85,-0.565685424949238));
#9706=CARTESIAN_POINT('',(-0.2,0.85,-0.39));
#9707=CARTESIAN_POINT('',(-0.2,0.,-0.565685424949238));
#9708=CARTESIAN_POINT('Origin',(0.2,-1.,-0.78));
#9709=CARTESIAN_POINT('',(0.2,-0.9,-0.78));
#9710=CARTESIAN_POINT('',(0.1,-0.9,-0.78));
#9711=CARTESIAN_POINT('',(0.2,0.85,-0.78));
#9712=CARTESIAN_POINT('',(0.2,-1.,-0.78));
#9713=CARTESIAN_POINT('',(0.1,0.85,-0.78));
#9714=CARTESIAN_POINT('',(-0.125,-0.5,-0.78));
#9715=CARTESIAN_POINT('Origin',(0.,-0.5,-0.78));
#9716=CARTESIAN_POINT('Origin',(0.2,-1.,0.));
#9717=CARTESIAN_POINT('',(0.2,-0.9,-0.565685424949238));
#9718=CARTESIAN_POINT('',(0.2,-0.9,0.));
#9719=CARTESIAN_POINT('',(0.2,0.85,-0.565685424949238));
#9720=CARTESIAN_POINT('',(0.2,0.,-0.565685424949238));
#9721=CARTESIAN_POINT('',(0.2,0.85,0.));
#9722=CARTESIAN_POINT('Origin',(0.,0.85,0.));
#9723=CARTESIAN_POINT('',(-1.4,0.85,1.71450551880629E-16));
#9724=CARTESIAN_POINT('Origin',(0.,0.85,0.));
#9725=CARTESIAN_POINT('Origin',(0.,0.85,0.));
#9726=CARTESIAN_POINT('Origin',(0.,0.,0.));
#9727=CARTESIAN_POINT('Origin',(0.,-0.9,0.));
#9728=CARTESIAN_POINT('',(0.125,-0.5,0.586834729715275));
#9729=CARTESIAN_POINT('',(-0.125,-0.5,0.586834729715275));
#9730=CARTESIAN_POINT('Ctrl Pts',(0.125,-0.5,0.586834729715275));
#9731=CARTESIAN_POINT('Ctrl Pts',(0.125,-0.484254474936005,0.586834729715275));
#9732=CARTESIAN_POINT('Ctrl Pts',(0.121843784097853,-0.467492086231842,
0.587534197873268));
#9733=CARTESIAN_POINT('Ctrl Pts',(0.109073016834181,-0.436709004341607,
0.590038488226116));
#9734=CARTESIAN_POINT('Ctrl Pts',(0.0994608796208941,-0.422684184324257,
0.591804743154611));
#9735=CARTESIAN_POINT('Ctrl Pts',(0.077316548567853,-0.400539853271216,
0.59510289473619));
#9736=CARTESIAN_POINT('Ctrl Pts',(0.0632914182239686,-0.390927142361291,
0.596852269967858));
#9737=CARTESIAN_POINT('Ctrl Pts',(0.0325072544867634,-0.378155958502111,
0.599317707212167));
#9738=CARTESIAN_POINT('Ctrl Pts',(0.0157444828659572,-0.375,0.6));
#9739=CARTESIAN_POINT('Ctrl Pts',(-0.0157444828659573,-0.375,0.6));
#9740=CARTESIAN_POINT('Ctrl Pts',(-0.0325072544867634,-0.378155958502111,
0.599317707212167));
#9741=CARTESIAN_POINT('Ctrl Pts',(-0.0632914182239687,-0.390927142361291,
0.596852269967858));
#9742=CARTESIAN_POINT('Ctrl Pts',(-0.077316548567853,-0.400539853271216,
0.59510289473619));
#9743=CARTESIAN_POINT('Ctrl Pts',(-0.0994608796208942,-0.422684184324257,
0.591804743154611));
#9744=CARTESIAN_POINT('Ctrl Pts',(-0.109073016834181,-0.436709004341607,
0.590038488226116));
#9745=CARTESIAN_POINT('Ctrl Pts',(-0.121843784097853,-0.467492086231842,
0.587534197873268));
#9746=CARTESIAN_POINT('Ctrl Pts',(-0.125,-0.484254474936005,0.586834729715275));
#9747=CARTESIAN_POINT('Ctrl Pts',(-0.125,-0.5,0.586834729715275));
#9748=CARTESIAN_POINT('Ctrl Pts',(-0.125,-0.5,0.586834729715275));
#9749=CARTESIAN_POINT('Ctrl Pts',(-0.125,-0.515745525063995,0.586834729715275));
#9750=CARTESIAN_POINT('Ctrl Pts',(-0.121843784097853,-0.532507913768158,
0.587534197873268));
#9751=CARTESIAN_POINT('Ctrl Pts',(-0.109073016834181,-0.563290995658393,
0.590038488226116));
#9752=CARTESIAN_POINT('Ctrl Pts',(-0.0994608796208941,-0.577315815675743,
0.591804743154611));
#9753=CARTESIAN_POINT('Ctrl Pts',(-0.077316548567853,-0.599460146728784,
0.59510289473619));
#9754=CARTESIAN_POINT('Ctrl Pts',(-0.0632914182239687,-0.609072857638709,
0.596852269967858));
#9755=CARTESIAN_POINT('Ctrl Pts',(-0.0325072544867635,-0.621844041497889,
0.599317707212167));
#9756=CARTESIAN_POINT('Ctrl Pts',(-0.0157444828659572,-0.625,0.6));
#9757=CARTESIAN_POINT('Ctrl Pts',(0.0157444828659572,-0.625,0.6));
#9758=CARTESIAN_POINT('Ctrl Pts',(0.0325072544867633,-0.621844041497889,
0.599317707212167));
#9759=CARTESIAN_POINT('Ctrl Pts',(0.0632914182239686,-0.609072857638709,
0.596852269967858));
#9760=CARTESIAN_POINT('Ctrl Pts',(0.077316548567853,-0.599460146728784,
0.59510289473619));
#9761=CARTESIAN_POINT('Ctrl Pts',(0.0994608796208942,-0.577315815675743,
0.591804743154611));
#9762=CARTESIAN_POINT('Ctrl Pts',(0.109073016834181,-0.563290995658393,
0.590038488226116));
#9763=CARTESIAN_POINT('Ctrl Pts',(0.121843784097853,-0.532507913768158,
0.587534197873268));
#9764=CARTESIAN_POINT('Ctrl Pts',(0.125,-0.515745525063995,0.586834729715275));
#9765=CARTESIAN_POINT('Ctrl Pts',(0.125,-0.5,0.586834729715275));
#9766=CARTESIAN_POINT('',(-0.586834729715275,-0.5,-0.125));
#9767=CARTESIAN_POINT('',(-0.586834729715275,-0.5,0.125));
#9768=CARTESIAN_POINT('Ctrl Pts',(-0.586834729715275,-0.5,-0.125));
#9769=CARTESIAN_POINT('Ctrl Pts',(-0.586834729715275,-0.515745525063995,
-0.125));
#9770=CARTESIAN_POINT('Ctrl Pts',(-0.587534197873268,-0.532507913768158,
-0.121843784097853));
#9771=CARTESIAN_POINT('Ctrl Pts',(-0.590038488226116,-0.563290995658393,
-0.109073016834181));
#9772=CARTESIAN_POINT('Ctrl Pts',(-0.591804743154611,-0.577315815675743,
-0.0994608796208942));
#9773=CARTESIAN_POINT('Ctrl Pts',(-0.59510289473619,-0.599460146728784,
-0.0773165485678531));
#9774=CARTESIAN_POINT('Ctrl Pts',(-0.596852269967858,-0.609072857638709,
-0.0632914182239687));
#9775=CARTESIAN_POINT('Ctrl Pts',(-0.599317707212167,-0.621844041497889,
-0.0325072544867635));
#9776=CARTESIAN_POINT('Ctrl Pts',(-0.6,-0.625,-0.0157444828659573));
#9777=CARTESIAN_POINT('Ctrl Pts',(-0.6,-0.625,0.0157444828659572));
#9778=CARTESIAN_POINT('Ctrl Pts',(-0.599317707212167,-0.621844041497889,
0.0325072544867633));
#9779=CARTESIAN_POINT('Ctrl Pts',(-0.596852269967858,-0.609072857638709,
0.0632914182239686));
#9780=CARTESIAN_POINT('Ctrl Pts',(-0.59510289473619,-0.599460146728784,
0.077316548567853));
#9781=CARTESIAN_POINT('Ctrl Pts',(-0.591804743154611,-0.577315815675743,
0.0994608796208941));
#9782=CARTESIAN_POINT('Ctrl Pts',(-0.590038488226116,-0.563290995658393,
0.109073016834181));
#9783=CARTESIAN_POINT('Ctrl Pts',(-0.587534197873268,-0.532507913768158,
0.121843784097853));
#9784=CARTESIAN_POINT('Ctrl Pts',(-0.586834729715275,-0.515745525063995,
0.125));
#9785=CARTESIAN_POINT('Ctrl Pts',(-0.586834729715275,-0.5,0.125));
#9786=CARTESIAN_POINT('Ctrl Pts',(-0.586834729715275,-0.5,0.125));
#9787=CARTESIAN_POINT('Ctrl Pts',(-0.586834729715275,-0.484254474936005,
0.125));
#9788=CARTESIAN_POINT('Ctrl Pts',(-0.587534197873268,-0.467492086231842,
0.121843784097853));
#9789=CARTESIAN_POINT('Ctrl Pts',(-0.590038488226116,-0.436709004341607,
0.109073016834181));
#9790=CARTESIAN_POINT('Ctrl Pts',(-0.591804743154611,-0.422684184324257,
0.0994608796208941));
#9791=CARTESIAN_POINT('Ctrl Pts',(-0.59510289473619,-0.400539853271216,
0.077316548567853));
#9792=CARTESIAN_POINT('Ctrl Pts',(-0.596852269967858,-0.390927142361291,
0.0632914182239686));
#9793=CARTESIAN_POINT('Ctrl Pts',(-0.599317707212167,-0.378155958502111,
0.0325072544867634));
#9794=CARTESIAN_POINT('Ctrl Pts',(-0.6,-0.375,0.0157444828659572));
#9795=CARTESIAN_POINT('Ctrl Pts',(-0.6,-0.375,-0.0157444828659572));
#9796=CARTESIAN_POINT('Ctrl Pts',(-0.599317707212167,-0.378155958502111,
-0.0325072544867634));
#9797=CARTESIAN_POINT('Ctrl Pts',(-0.596852269967858,-0.390927142361291,
-0.0632914182239686));
#9798=CARTESIAN_POINT('Ctrl Pts',(-0.59510289473619,-0.400539853271216,
-0.077316548567853));
#9799=CARTESIAN_POINT('Ctrl Pts',(-0.591804743154611,-0.422684184324257,
-0.0994608796208942));
#9800=CARTESIAN_POINT('Ctrl Pts',(-0.590038488226116,-0.436709004341607,
-0.109073016834181));
#9801=CARTESIAN_POINT('Ctrl Pts',(-0.587534197873268,-0.467492086231842,
-0.121843784097853));
#9802=CARTESIAN_POINT('Ctrl Pts',(-0.586834729715275,-0.484254474936005,
-0.125));
#9803=CARTESIAN_POINT('Ctrl Pts',(-0.586834729715275,-0.5,-0.125));
#9804=CARTESIAN_POINT('',(0.586834729715275,-0.5,-0.125));
#9805=CARTESIAN_POINT('',(0.586834729715275,-0.5,0.125));
#9806=CARTESIAN_POINT('Ctrl Pts',(0.586834729715275,-0.5,-0.125));
#9807=CARTESIAN_POINT('Ctrl Pts',(0.586834729715275,-0.484254474936005,
-0.125));
#9808=CARTESIAN_POINT('Ctrl Pts',(0.587534197873268,-0.467492086231842,
-0.121843784097853));
#9809=CARTESIAN_POINT('Ctrl Pts',(0.590038488226116,-0.436709004341607,
-0.109073016834181));
#9810=CARTESIAN_POINT('Ctrl Pts',(0.591804743154611,-0.422684184324257,
-0.0994608796208941));
#9811=CARTESIAN_POINT('Ctrl Pts',(0.59510289473619,-0.400539853271216,-0.0773165485678529));
#9812=CARTESIAN_POINT('Ctrl Pts',(0.596852269967858,-0.390927142361291,
-0.0632914182239686));
#9813=CARTESIAN_POINT('Ctrl Pts',(0.599317707212167,-0.378155958502111,
-0.0325072544867633));
#9814=CARTESIAN_POINT('Ctrl Pts',(0.6,-0.375,-0.0157444828659572));
#9815=CARTESIAN_POINT('Ctrl Pts',(0.6,-0.375,0.0157444828659573));
#9816=CARTESIAN_POINT('Ctrl Pts',(0.599317707212167,-0.378155958502111,
0.0325072544867635));
#9817=CARTESIAN_POINT('Ctrl Pts',(0.596852269967858,-0.390927142361291,
0.0632914182239687));
#9818=CARTESIAN_POINT('Ctrl Pts',(0.59510289473619,-0.400539853271216,0.0773165485678531));
#9819=CARTESIAN_POINT('Ctrl Pts',(0.591804743154611,-0.422684184324257,
0.0994608796208942));
#9820=CARTESIAN_POINT('Ctrl Pts',(0.590038488226116,-0.436709004341607,
0.109073016834181));
#9821=CARTESIAN_POINT('Ctrl Pts',(0.587534197873268,-0.467492086231842,
0.121843784097853));
#9822=CARTESIAN_POINT('Ctrl Pts',(0.586834729715275,-0.484254474936005,
0.125));
#9823=CARTESIAN_POINT('Ctrl Pts',(0.586834729715275,-0.5,0.125));
#9824=CARTESIAN_POINT('Ctrl Pts',(0.586834729715275,-0.5,0.125));
#9825=CARTESIAN_POINT('Ctrl Pts',(0.586834729715275,-0.515745525063995,
0.125));
#9826=CARTESIAN_POINT('Ctrl Pts',(0.587534197873268,-0.532507913768158,
0.121843784097853));
#9827=CARTESIAN_POINT('Ctrl Pts',(0.590038488226116,-0.563290995658393,
0.109073016834181));
#9828=CARTESIAN_POINT('Ctrl Pts',(0.591804743154611,-0.577315815675743,
0.0994608796208942));
#9829=CARTESIAN_POINT('Ctrl Pts',(0.59510289473619,-0.599460146728784,0.077316548567853));
#9830=CARTESIAN_POINT('Ctrl Pts',(0.596852269967858,-0.609072857638709,
0.0632914182239688));
#9831=CARTESIAN_POINT('Ctrl Pts',(0.599317707212167,-0.621844041497889,
0.0325072544867635));
#9832=CARTESIAN_POINT('Ctrl Pts',(0.6,-0.625,0.0157444828659573));
#9833=CARTESIAN_POINT('Ctrl Pts',(0.6,-0.625,-0.0157444828659572));
#9834=CARTESIAN_POINT('Ctrl Pts',(0.599317707212167,-0.621844041497889,
-0.0325072544867633));
#9835=CARTESIAN_POINT('Ctrl Pts',(0.596852269967858,-0.609072857638709,
-0.0632914182239685));
#9836=CARTESIAN_POINT('Ctrl Pts',(0.59510289473619,-0.599460146728784,-0.077316548567853));
#9837=CARTESIAN_POINT('Ctrl Pts',(0.591804743154611,-0.577315815675743,
-0.0994608796208941));
#9838=CARTESIAN_POINT('Ctrl Pts',(0.590038488226116,-0.563290995658393,
-0.10907301683418));
#9839=CARTESIAN_POINT('Ctrl Pts',(0.587534197873268,-0.532507913768158,
-0.121843784097853));
#9840=CARTESIAN_POINT('Ctrl Pts',(0.586834729715275,-0.515745525063995,
-0.125));
#9841=CARTESIAN_POINT('Ctrl Pts',(0.586834729715275,-0.5,-0.125));
#9842=CARTESIAN_POINT('Origin',(0.,-0.5,0.));
#9843=CARTESIAN_POINT('',(-1.,-0.375,-6.12323399573677E-17));
#9844=CARTESIAN_POINT('',(-0.992156741649222,-0.5,0.125));
#9845=CARTESIAN_POINT('Ctrl Pts',(-1.,-0.375,-1.00613961606655E-16));
#9846=CARTESIAN_POINT('Ctrl Pts',(-1.,-0.375,0.0157128711428661));
#9847=CARTESIAN_POINT('Ctrl Pts',(-0.999591823858855,-0.378143583103513,
0.0324619190698278));
#9848=CARTESIAN_POINT('Ctrl Pts',(-0.998116453123232,-0.390905426591754,
0.0632545375991437));
#9849=CARTESIAN_POINT('Ctrl Pts',(-0.997070068816062,-0.400522781657727,
0.0772994769543643));
#9850=CARTESIAN_POINT('Ctrl Pts',(-0.995102104277285,-0.422700615683787,
0.0994773109804239));
#9851=CARTESIAN_POINT('Ctrl Pts',(-0.994052129228928,-0.436745514765346,
0.109094593469654));
#9852=CARTESIAN_POINT('Ctrl Pts',(-0.99256853061881,-0.467537996927464,
0.121856383722779));
#9853=CARTESIAN_POINT('Ctrl Pts',(-0.992156741649222,-0.484286997589363,
0.125));
#9854=CARTESIAN_POINT('Ctrl Pts',(-0.992156741649222,-0.5,0.125));
#9855=CARTESIAN_POINT('',(-1.,-0.625,-6.12323399573677E-17));
#9856=CARTESIAN_POINT('Ctrl Pts',(-1.,-0.625,-4.5102810375397E-17));
#9857=CARTESIAN_POINT('Ctrl Pts',(-1.,-0.625,-0.0157128711428662));
#9858=CARTESIAN_POINT('Ctrl Pts',(-0.999591823858855,-0.621856416896487,
-0.032461919069828));
#9859=CARTESIAN_POINT('Ctrl Pts',(-0.998116453123232,-0.609094573408246,
-0.0632545375991439));
#9860=CARTESIAN_POINT('Ctrl Pts',(-0.997070068816062,-0.599477218342273,
-0.0772994769543645));
#9861=CARTESIAN_POINT('Ctrl Pts',(-0.995102104277285,-0.577299384316213,
-0.0994773109804241));
#9862=CARTESIAN_POINT('Ctrl Pts',(-0.994052129228928,-0.563254485234654,
-0.109094593469655));
#9863=CARTESIAN_POINT('Ctrl Pts',(-0.99256853061881,-0.532462003072536,
-0.121856383722779));
#9864=CARTESIAN_POINT('Ctrl Pts',(-0.992156741649221,-0.515713002410637,
-0.125));
#9865=CARTESIAN_POINT('Ctrl Pts',(-0.992156741649221,-0.484286997589363,
-0.125));
#9866=CARTESIAN_POINT('Ctrl Pts',(-0.99256853061881,-0.467537996927464,
-0.121856383722779));
#9867=CARTESIAN_POINT('Ctrl Pts',(-0.994052129228928,-0.436745514765346,
-0.109094593469655));
#9868=CARTESIAN_POINT('Ctrl Pts',(-0.995102104277285,-0.422700615683787,
-0.0994773109804241));
#9869=CARTESIAN_POINT('Ctrl Pts',(-0.997070068816062,-0.400522781657728,
-0.0772994769543645));
#9870=CARTESIAN_POINT('Ctrl Pts',(-0.998116453123232,-0.390905426591754,
-0.063254537599144));
#9871=CARTESIAN_POINT('Ctrl Pts',(-0.999591823858855,-0.378143583103513,
-0.0324619190698281));
#9872=CARTESIAN_POINT('Ctrl Pts',(-1.,-0.375,-0.0157128711428663));
#9873=CARTESIAN_POINT('Ctrl Pts',(-1.,-0.375,-9.36750677027476E-17));
#9874=CARTESIAN_POINT('Ctrl Pts',(-0.992156741649222,-0.5,0.125));
#9875=CARTESIAN_POINT('Ctrl Pts',(-0.992156741649222,-0.515713002410637,
0.125));
#9876=CARTESIAN_POINT('Ctrl Pts',(-0.99256853061881,-0.532462003072536,
0.121856383722779));
#9877=CARTESIAN_POINT('Ctrl Pts',(-0.994052129228928,-0.563254485234654,
0.109094593469654));
#9878=CARTESIAN_POINT('Ctrl Pts',(-0.995102104277285,-0.577299384316213,
0.0994773109804241));
#9879=CARTESIAN_POINT('Ctrl Pts',(-0.997070068816062,-0.599477218342273,
0.0772994769543644));
#9880=CARTESIAN_POINT('Ctrl Pts',(-0.998116453123232,-0.609094573408246,
0.0632545375991438));
#9881=CARTESIAN_POINT('Ctrl Pts',(-0.999591823858855,-0.621856416896487,
0.0324619190698279));
#9882=CARTESIAN_POINT('Ctrl Pts',(-1.,-0.625,0.0157128711428661));
#9883=CARTESIAN_POINT('Ctrl Pts',(-1.,-0.625,-4.85722573273506E-17));
#9884=CARTESIAN_POINT('',(-7.65404249467096E-18,-0.5,0.125));
#9885=CARTESIAN_POINT('Origin',(0.,-0.5,0.));
#9886=CARTESIAN_POINT('',(0.992156741649222,-0.5,0.125));
#9887=CARTESIAN_POINT('',(-7.65404249467096E-18,-0.5,0.125));
#9888=CARTESIAN_POINT('',(1.,-0.625,6.12323399573677E-17));
#9889=CARTESIAN_POINT('Ctrl Pts',(1.,-0.625,7.28583859910259E-17));
#9890=CARTESIAN_POINT('Ctrl Pts',(1.,-0.625,0.0157128711428663));
#9891=CARTESIAN_POINT('Ctrl Pts',(0.999591823858855,-0.621856416896487,
0.032461919069828));
#9892=CARTESIAN_POINT('Ctrl Pts',(0.998116453123232,-0.609094573408246,
0.0632545375991439));
#9893=CARTESIAN_POINT('Ctrl Pts',(0.997070068816062,-0.599477218342273,
0.0772994769543645));
#9894=CARTESIAN_POINT('Ctrl Pts',(0.995102104277285,-0.577299384316213,
0.0994773109804242));
#9895=CARTESIAN_POINT('Ctrl Pts',(0.994052129228928,-0.563254485234654,
0.109094593469655));
#9896=CARTESIAN_POINT('Ctrl Pts',(0.99256853061881,-0.532462003072536,0.121856383722779));
#9897=CARTESIAN_POINT('Ctrl Pts',(0.992156741649222,-0.515713002410637,
0.125));
#9898=CARTESIAN_POINT('Ctrl Pts',(0.992156741649222,-0.5,0.125));
#9899=CARTESIAN_POINT('',(1.,-0.375,6.12323399573677E-17));
#9900=CARTESIAN_POINT('Ctrl Pts',(1.,-0.375,2.08166817117217E-17));
#9901=CARTESIAN_POINT('Ctrl Pts',(1.,-0.375,-0.0157128711428662));
#9902=CARTESIAN_POINT('Ctrl Pts',(0.999591823858855,-0.378143583103513,
-0.032461919069828));
#9903=CARTESIAN_POINT('Ctrl Pts',(0.998116453123232,-0.390905426591754,
-0.0632545375991438));
#9904=CARTESIAN_POINT('Ctrl Pts',(0.997070068816062,-0.400522781657728,
-0.0772994769543644));
#9905=CARTESIAN_POINT('Ctrl Pts',(0.995102104277285,-0.422700615683787,
-0.099477310980424));
#9906=CARTESIAN_POINT('Ctrl Pts',(0.994052129228928,-0.436745514765346,
-0.109094593469654));
#9907=CARTESIAN_POINT('Ctrl Pts',(0.99256853061881,-0.467537996927464,-0.121856383722779));
#9908=CARTESIAN_POINT('Ctrl Pts',(0.992156741649222,-0.484286997589363,
-0.125));
#9909=CARTESIAN_POINT('Ctrl Pts',(0.992156741649222,-0.515713002410637,
-0.125));
#9910=CARTESIAN_POINT('Ctrl Pts',(0.99256853061881,-0.532462003072536,-0.121856383722779));
#9911=CARTESIAN_POINT('Ctrl Pts',(0.994052129228928,-0.563254485234654,
-0.109094593469654));
#9912=CARTESIAN_POINT('Ctrl Pts',(0.995102104277285,-0.577299384316213,
-0.099477310980424));
#9913=CARTESIAN_POINT('Ctrl Pts',(0.997070068816062,-0.599477218342273,
-0.0772994769543643));
#9914=CARTESIAN_POINT('Ctrl Pts',(0.998116453123232,-0.609094573408246,
-0.0632545375991438));
#9915=CARTESIAN_POINT('Ctrl Pts',(0.999591823858855,-0.621856416896487,
-0.0324619190698279));
#9916=CARTESIAN_POINT('Ctrl Pts',(1.,-0.625,-0.0157128711428661));
#9917=CARTESIAN_POINT('Ctrl Pts',(1.,-0.625,8.32667268468867E-17));
#9918=CARTESIAN_POINT('Ctrl Pts',(0.992156741649222,-0.5,0.125));
#9919=CARTESIAN_POINT('Ctrl Pts',(0.992156741649222,-0.484286997589363,
0.125));
#9920=CARTESIAN_POINT('Ctrl Pts',(0.99256853061881,-0.467537996927464,0.121856383722779));
#9921=CARTESIAN_POINT('Ctrl Pts',(0.994052129228928,-0.436745514765346,
0.109094593469654));
#9922=CARTESIAN_POINT('Ctrl Pts',(0.995102104277285,-0.422700615683787,
0.0994773109804241));
#9923=CARTESIAN_POINT('Ctrl Pts',(0.997070068816062,-0.400522781657727,
0.0772994769543644));
#9924=CARTESIAN_POINT('Ctrl Pts',(0.998116453123232,-0.390905426591754,
0.0632545375991438));
#9925=CARTESIAN_POINT('Ctrl Pts',(0.999591823858855,-0.378143583103513,
0.0324619190698279));
#9926=CARTESIAN_POINT('Ctrl Pts',(1.,-0.375,0.0157128711428662));
#9927=CARTESIAN_POINT('Ctrl Pts',(1.,-0.375,2.77555756156289E-17));
#9928=CARTESIAN_POINT('Origin',(0.,-0.1,0.));
#9929=CARTESIAN_POINT('',(-1.,-0.9,1.22464679914735E-16));
#9930=CARTESIAN_POINT('Origin',(0.,-0.9,0.));
#9931=CARTESIAN_POINT('',(-1.,-0.1,-1.22464679914735E-16));
#9932=CARTESIAN_POINT('',(-1.,-0.1,1.22464679914735E-16));
#9933=CARTESIAN_POINT('',(-1.,-0.1,-1.22464679914735E-16));
#9934=CARTESIAN_POINT('Origin',(0.,-0.1,0.));
#9935=CARTESIAN_POINT('',(0.,-0.625,-1.));
#9936=CARTESIAN_POINT('',(0.,-0.375,-1.));
#9937=CARTESIAN_POINT('Ctrl Pts',(-2.08166817117217E-17,-0.625,-1.));
#9938=CARTESIAN_POINT('Ctrl Pts',(0.0157128711428662,-0.625,-1.));
#9939=CARTESIAN_POINT('Ctrl Pts',(0.0324619190698279,-0.621856416896487,
-0.999591823858855));
#9940=CARTESIAN_POINT('Ctrl Pts',(0.0632545375991438,-0.609094573408246,
-0.998116453123232));
#9941=CARTESIAN_POINT('Ctrl Pts',(0.0772994769543644,-0.599477218342273,
-0.997070068816062));
#9942=CARTESIAN_POINT('Ctrl Pts',(0.0994773109804241,-0.577299384316213,
-0.995102104277285));
#9943=CARTESIAN_POINT('Ctrl Pts',(0.109094593469654,-0.563254485234654,
-0.994052129228928));
#9944=CARTESIAN_POINT('Ctrl Pts',(0.121856383722779,-0.532462003072536,
-0.99256853061881));
#9945=CARTESIAN_POINT('Ctrl Pts',(0.125,-0.515713002410637,-0.992156741649221));
#9946=CARTESIAN_POINT('Ctrl Pts',(0.125,-0.484286997589363,-0.992156741649221));
#9947=CARTESIAN_POINT('Ctrl Pts',(0.121856383722779,-0.467537996927464,
-0.99256853061881));
#9948=CARTESIAN_POINT('Ctrl Pts',(0.109094593469654,-0.436745514765346,
-0.994052129228928));
#9949=CARTESIAN_POINT('Ctrl Pts',(0.0994773109804241,-0.422700615683787,
-0.995102104277285));
#9950=CARTESIAN_POINT('Ctrl Pts',(0.0772994769543645,-0.400522781657728,
-0.997070068816062));
#9951=CARTESIAN_POINT('Ctrl Pts',(0.0632545375991439,-0.390905426591754,
-0.998116453123232));
#9952=CARTESIAN_POINT('Ctrl Pts',(0.032461919069828,-0.378143583103513,
-0.999591823858855));
#9953=CARTESIAN_POINT('Ctrl Pts',(0.0157128711428662,-0.375,-1.));
#9954=CARTESIAN_POINT('Ctrl Pts',(3.81639164714898E-17,-0.375,-1.));
#9955=CARTESIAN_POINT('',(-0.125,-0.5,-0.992156741649222));
#9956=CARTESIAN_POINT('Ctrl Pts',(4.5102810375397E-17,-0.375,-1.));
#9957=CARTESIAN_POINT('Ctrl Pts',(-0.0157128711428661,-0.375,-1.));
#9958=CARTESIAN_POINT('Ctrl Pts',(-0.0324619190698279,-0.378143583103513,
-0.999591823858855));
#9959=CARTESIAN_POINT('Ctrl Pts',(-0.0632545375991437,-0.390905426591754,
-0.998116453123232));
#9960=CARTESIAN_POINT('Ctrl Pts',(-0.0772994769543643,-0.400522781657727,
-0.997070068816062));
#9961=CARTESIAN_POINT('Ctrl Pts',(-0.099477310980424,-0.422700615683787,
-0.995102104277285));
#9962=CARTESIAN_POINT('Ctrl Pts',(-0.109094593469654,-0.436745514765346,
-0.994052129228928));
#9963=CARTESIAN_POINT('Ctrl Pts',(-0.121856383722779,-0.467537996927464,
-0.99256853061881));
#9964=CARTESIAN_POINT('Ctrl Pts',(-0.125,-0.484286997589363,-0.992156741649222));
#9965=CARTESIAN_POINT('Ctrl Pts',(-0.125,-0.5,-0.992156741649222));
#9966=CARTESIAN_POINT('Ctrl Pts',(-0.125,-0.5,-0.992156741649222));
#9967=CARTESIAN_POINT('Ctrl Pts',(-0.125,-0.515713002410637,-0.992156741649222));
#9968=CARTESIAN_POINT('Ctrl Pts',(-0.121856383722779,-0.532462003072536,
-0.99256853061881));
#9969=CARTESIAN_POINT('Ctrl Pts',(-0.109094593469654,-0.563254485234654,
-0.994052129228928));
#9970=CARTESIAN_POINT('Ctrl Pts',(-0.0994773109804241,-0.577299384316213,
-0.995102104277285));
#9971=CARTESIAN_POINT('Ctrl Pts',(-0.0772994769543644,-0.599477218342273,
-0.997070068816062));
#9972=CARTESIAN_POINT('Ctrl Pts',(-0.0632545375991439,-0.609094573408246,
-0.998116453123232));
#9973=CARTESIAN_POINT('Ctrl Pts',(-0.032461919069828,-0.621856416896487,
-0.999591823858855));
#9974=CARTESIAN_POINT('Ctrl Pts',(-0.0157128711428662,-0.625,-1.));
#9975=CARTESIAN_POINT('Ctrl Pts',(-1.38777878078145E-17,-0.625,-1.));
#9976=CARTESIAN_POINT('',(0.,-0.375,1.));
#9977=CARTESIAN_POINT('',(0.,-0.625,1.));
#9978=CARTESIAN_POINT('Ctrl Pts',(4.16333634234434E-17,-0.375,1.));
#9979=CARTESIAN_POINT('Ctrl Pts',(0.0157128711428662,-0.375,1.));
#9980=CARTESIAN_POINT('Ctrl Pts',(0.032461919069828,-0.378143583103513,
0.999591823858855));
#9981=CARTESIAN_POINT('Ctrl Pts',(0.0632545375991439,-0.390905426591754,
0.998116453123232));
#9982=CARTESIAN_POINT('Ctrl Pts',(0.0772994769543644,-0.400522781657728,
0.997070068816062));
#9983=CARTESIAN_POINT('Ctrl Pts',(0.0994773109804241,-0.422700615683787,
0.995102104277285));
#9984=CARTESIAN_POINT('Ctrl Pts',(0.109094593469654,-0.436745514765346,
0.994052129228928));
#9985=CARTESIAN_POINT('Ctrl Pts',(0.121856383722779,-0.467537996927464,
0.99256853061881));
#9986=CARTESIAN_POINT('Ctrl Pts',(0.125,-0.484286997589363,0.992156741649222));
#9987=CARTESIAN_POINT('Ctrl Pts',(0.125,-0.515713002410637,0.992156741649222));
#9988=CARTESIAN_POINT('Ctrl Pts',(0.121856383722779,-0.532462003072536,
0.99256853061881));
#9989=CARTESIAN_POINT('Ctrl Pts',(0.109094593469655,-0.563254485234654,
0.994052129228928));
#9990=CARTESIAN_POINT('Ctrl Pts',(0.0994773109804241,-0.577299384316213,
0.995102104277285));
#9991=CARTESIAN_POINT('Ctrl Pts',(0.0772994769543644,-0.599477218342273,
0.997070068816062));
#9992=CARTESIAN_POINT('Ctrl Pts',(0.0632545375991438,-0.609094573408246,
0.998116453123232));
#9993=CARTESIAN_POINT('Ctrl Pts',(0.0324619190698279,-0.621856416896487,
0.999591823858855));
#9994=CARTESIAN_POINT('Ctrl Pts',(0.0157128711428662,-0.625,1.));
#9995=CARTESIAN_POINT('Ctrl Pts',(-1.73472347597681E-17,-0.625,1.));
#9996=CARTESIAN_POINT('',(-0.125,-0.5,0.992156741649222));
#9997=CARTESIAN_POINT('Ctrl Pts',(-1.73472347597681E-17,-0.625,1.));
#9998=CARTESIAN_POINT('Ctrl Pts',(-0.0157128711428662,-0.625,1.));
#9999=CARTESIAN_POINT('Ctrl Pts',(-0.032461919069828,-0.621856416896487,
0.999591823858855));
#10000=CARTESIAN_POINT('Ctrl Pts',(-0.0632545375991439,-0.609094573408246,
0.998116453123232));
#10001=CARTESIAN_POINT('Ctrl Pts',(-0.0772994769543645,-0.599477218342273,
0.997070068816062));
#10002=CARTESIAN_POINT('Ctrl Pts',(-0.0994773109804241,-0.577299384316213,
0.995102104277285));
#10003=CARTESIAN_POINT('Ctrl Pts',(-0.109094593469654,-0.563254485234654,
0.994052129228928));
#10004=CARTESIAN_POINT('Ctrl Pts',(-0.121856383722779,-0.532462003072536,
0.99256853061881));
#10005=CARTESIAN_POINT('Ctrl Pts',(-0.125,-0.515713002410637,0.992156741649222));
#10006=CARTESIAN_POINT('Ctrl Pts',(-0.125,-0.5,0.992156741649222));
#10007=CARTESIAN_POINT('Ctrl Pts',(-0.125,-0.5,0.992156741649222));
#10008=CARTESIAN_POINT('Ctrl Pts',(-0.125,-0.484286997589363,0.992156741649222));
#10009=CARTESIAN_POINT('Ctrl Pts',(-0.121856383722779,-0.467537996927464,
0.99256853061881));
#10010=CARTESIAN_POINT('Ctrl Pts',(-0.109094593469654,-0.436745514765346,
0.994052129228928));
#10011=CARTESIAN_POINT('Ctrl Pts',(-0.099477310980424,-0.422700615683787,
0.995102104277285));
#10012=CARTESIAN_POINT('Ctrl Pts',(-0.0772994769543643,-0.400522781657727,
0.997070068816062));
#10013=CARTESIAN_POINT('Ctrl Pts',(-0.0632545375991438,-0.390905426591754,
0.998116453123232));
#10014=CARTESIAN_POINT('Ctrl Pts',(-0.0324619190698279,-0.378143583103513,
0.999591823858855));
#10015=CARTESIAN_POINT('Ctrl Pts',(-0.0157128711428661,-0.375,1.));
#10016=CARTESIAN_POINT('Ctrl Pts',(4.5102810375397E-17,-0.375,1.));
#10017=CARTESIAN_POINT('Origin',(0.,-0.5,0.));
#10018=CARTESIAN_POINT('',(-0.125,-0.5,0.));
#10019=CARTESIAN_POINT('Origin',(0.,-0.5,0.));
#10020=CARTESIAN_POINT('',(-0.125,-0.5,0.));
#10021=CARTESIAN_POINT('Origin',(0.,-0.9,0.));
#10022=CARTESIAN_POINT('Origin',(0.,0.,0.));
#10023=CARTESIAN_POINT('',(-1.4,0.,1.71450551880629E-16));
#10024=CARTESIAN_POINT('Origin',(0.,0.,0.));
#10025=CARTESIAN_POINT('',(1.23958209161204,0.,0.143317017690053));
#10026=CARTESIAN_POINT('',(1.22320001975977,0.,0.246749348660852));
#10027=CARTESIAN_POINT('Origin',(1.21321664662686,0.,0.192154639568406));
#10028=CARTESIAN_POINT('',(1.20190105810224,0.,0.335465908756113));
#10029=CARTESIAN_POINT('Origin',(0.,0.,0.));
#10030=CARTESIAN_POINT('',(1.16954029537568,0.,0.435062095450087));
#10031=CARTESIAN_POINT('Origin',(1.1682203282434,0.,0.379577794185952));
#10032=CARTESIAN_POINT('',(1.13462523166105,0.,0.519354515801077));
#10033=CARTESIAN_POINT('Origin',(0.,0.,0.));
#10034=CARTESIAN_POINT('',(1.08708260743774,0.,0.612662169561029));
#10035=CARTESIAN_POINT('Origin',(1.0944585482776,0.,0.557654483764164));
#10036=CARTESIAN_POINT('',(1.0394111664111,0.,0.690454891028201));
#10037=CARTESIAN_POINT('Origin',(0.,0.,0.));
#10038=CARTESIAN_POINT('',(0.977857337884349,0.,0.775176467748211));
#10039=CARTESIAN_POINT('Origin',(0.993747566553533,0.,0.72199986920298));
#10040=CARTESIAN_POINT('',(0.918603348636233,0.,0.844553975349804));
#10041=CARTESIAN_POINT('Origin',(0.,0.,0.));
#10042=CARTESIAN_POINT('',(0.844553975349804,0.,0.918603348636233));
#10043=CARTESIAN_POINT('Origin',(0.86856722168183,0.,0.86856722168183));
#10044=CARTESIAN_POINT('',(0.775176467748211,0.,0.977857337884349));
#10045=CARTESIAN_POINT('Origin',(0.,0.,0.));
#10046=CARTESIAN_POINT('',(0.690454891028201,0.,1.0394111664111));
#10047=CARTESIAN_POINT('Origin',(0.721999869202979,0.,0.993747566553533));
#10048=CARTESIAN_POINT('',(0.612662169561028,0.,1.08708260743774));
#10049=CARTESIAN_POINT('Origin',(0.,0.,0.));
#10050=CARTESIAN_POINT('',(0.519354515801077,0.,1.13462523166105));
#10051=CARTESIAN_POINT('Origin',(0.557654483764164,0.,1.0944585482776));
#10052=CARTESIAN_POINT('',(0.435062095450087,0.,1.16954029537568));
#10053=CARTESIAN_POINT('Origin',(0.,0.,0.));
#10054=CARTESIAN_POINT('',(0.335465908756113,0.,1.20190105810224));
#10055=CARTESIAN_POINT('Origin',(0.379577794185951,0.,1.1682203282434));
#10056=CARTESIAN_POINT('',(0.246749348660851,0.,1.22320001975977));
#10057=CARTESIAN_POINT('Origin',(0.,0.,0.));
#10058=CARTESIAN_POINT('',(0.143317017690053,0.,1.23958209161204));
#10059=CARTESIAN_POINT('Origin',(0.192154639568406,0.,1.21321664662686));
#10060=CARTESIAN_POINT('',(0.0523608139934478,0.,1.24674050008925));
#10061=CARTESIAN_POINT('Origin',(0.,0.,0.));
#10062=CARTESIAN_POINT('',(-0.0523608139934483,0.,1.24674050008925));
#10063=CARTESIAN_POINT('Origin',(-2.25642313758905E-16,0.,1.22833954473516));
#10064=CARTESIAN_POINT('',(-0.143317017690053,0.,1.23958209161204));
#10065=CARTESIAN_POINT('Origin',(0.,0.,0.));
#10066=CARTESIAN_POINT('',(-0.246749348660852,0.,1.22320001975977));
#10067=CARTESIAN_POINT('Origin',(-0.192154639568406,0.,1.21321664662686));
#10068=CARTESIAN_POINT('',(-0.335465908756113,0.,1.20190105810224));
#10069=CARTESIAN_POINT('Origin',(0.,0.,0.));
#10070=CARTESIAN_POINT('',(-0.435062095450087,0.,1.16954029537568));
#10071=CARTESIAN_POINT('Origin',(-0.379577794185951,0.,1.1682203282434));
#10072=CARTESIAN_POINT('',(-0.519354515801077,0.,1.13462523166105));
#10073=CARTESIAN_POINT('Origin',(0.,0.,0.));
#10074=CARTESIAN_POINT('',(-0.612662169561029,0.,1.08708260743774));
#10075=CARTESIAN_POINT('Origin',(-0.557654483764164,0.,1.0944585482776));
#10076=CARTESIAN_POINT('',(-0.690454891028201,0.,1.0394111664111));
#10077=CARTESIAN_POINT('Origin',(0.,0.,0.));
#10078=CARTESIAN_POINT('',(-0.775176467748211,0.,0.977857337884349));
#10079=CARTESIAN_POINT('Origin',(-0.721999869202979,0.,0.993747566553533));
#10080=CARTESIAN_POINT('',(-0.844553975349804,0.,0.918603348636233));
#10081=CARTESIAN_POINT('Origin',(0.,0.,0.));
#10082=CARTESIAN_POINT('',(-0.918603348636233,0.,0.844553975349804));
#10083=CARTESIAN_POINT('Origin',(-0.86856722168183,0.,0.86856722168183));
#10084=CARTESIAN_POINT('',(-0.977857337884348,0.,0.775176467748211));
#10085=CARTESIAN_POINT('Origin',(0.,0.,0.));
#10086=CARTESIAN_POINT('',(-1.0394111664111,0.,0.690454891028201));
#10087=CARTESIAN_POINT('Origin',(-0.993747566553533,0.,0.721999869202979));
#10088=CARTESIAN_POINT('',(-1.08708260743774,0.,0.612662169561028));
#10089=CARTESIAN_POINT('Origin',(0.,0.,0.));
#10090=CARTESIAN_POINT('',(-1.13462523166105,0.,0.519354515801077));
#10091=CARTESIAN_POINT('Origin',(-1.0944585482776,0.,0.557654483764164));
#10092=CARTESIAN_POINT('',(-1.16954029537568,0.,0.435062095450087));
#10093=CARTESIAN_POINT('Origin',(0.,0.,0.));
#10094=CARTESIAN_POINT('',(-1.20190105810224,0.,0.335465908756113));
#10095=CARTESIAN_POINT('Origin',(-1.1682203282434,0.,0.379577794185951));
#10096=CARTESIAN_POINT('',(-1.22320001975977,0.,0.246749348660851));
#10097=CARTESIAN_POINT('Origin',(0.,0.,0.));
#10098=CARTESIAN_POINT('',(-1.23958209161204,0.,0.143317017690053));
#10099=CARTESIAN_POINT('Origin',(-1.21321664662686,0.,0.192154639568406));
#10100=CARTESIAN_POINT('',(-1.24674050008925,0.,0.0523608139934479));
#10101=CARTESIAN_POINT('Origin',(0.,0.,0.));
#10102=CARTESIAN_POINT('',(-1.24674050008925,0.,-0.0523608139934482));
#10103=CARTESIAN_POINT('Origin',(-1.22833954473516,0.,-1.50428209172603E-16));
#10104=CARTESIAN_POINT('',(-1.23958209161204,0.,-0.143317017690053));
#10105=CARTESIAN_POINT('Origin',(0.,0.,0.));
#10106=CARTESIAN_POINT('',(-1.22320001975977,0.,-0.246749348660852));
#10107=CARTESIAN_POINT('Origin',(-1.21321664662686,0.,-0.192154639568406));
#10108=CARTESIAN_POINT('',(-1.20190105810224,0.,-0.335465908756113));
#10109=CARTESIAN_POINT('Origin',(0.,0.,0.));
#10110=CARTESIAN_POINT('',(-1.16954029537568,0.,-0.435062095450087));
#10111=CARTESIAN_POINT('Origin',(-1.1682203282434,0.,-0.379577794185951));
#10112=CARTESIAN_POINT('',(-1.13462523166105,0.,-0.519354515801077));
#10113=CARTESIAN_POINT('Origin',(0.,0.,0.));
#10114=CARTESIAN_POINT('',(-1.08708260743774,0.,-0.612662169561029));
#10115=CARTESIAN_POINT('Origin',(-1.0944585482776,0.,-0.557654483764164));
#10116=CARTESIAN_POINT('',(-1.0394111664111,0.,-0.690454891028201));
#10117=CARTESIAN_POINT('Origin',(0.,0.,0.));
#10118=CARTESIAN_POINT('',(-0.977857337884349,0.,-0.775176467748211));
#10119=CARTESIAN_POINT('Origin',(-0.993747566553533,0.,-0.721999869202979));
#10120=CARTESIAN_POINT('',(-0.918603348636233,0.,-0.844553975349804));
#10121=CARTESIAN_POINT('Origin',(0.,0.,0.));
#10122=CARTESIAN_POINT('',(-0.844553975349804,0.,-0.918603348636233));
#10123=CARTESIAN_POINT('Origin',(-0.86856722168183,0.,-0.86856722168183));
#10124=CARTESIAN_POINT('',(-0.775176467748211,0.,-0.977857337884348));
#10125=CARTESIAN_POINT('Origin',(0.,0.,0.));
#10126=CARTESIAN_POINT('',(-0.690454891028201,0.,-1.0394111664111));
#10127=CARTESIAN_POINT('Origin',(-0.721999869202979,0.,-0.993747566553533));
#10128=CARTESIAN_POINT('',(-0.612662169561028,0.,-1.08708260743774));
#10129=CARTESIAN_POINT('Origin',(0.,0.,0.));
#10130=CARTESIAN_POINT('',(-0.519354515801077,0.,-1.13462523166105));
#10131=CARTESIAN_POINT('Origin',(-0.557654483764164,0.,-1.0944585482776));
#10132=CARTESIAN_POINT('',(-0.435062095450087,0.,-1.16954029537568));
#10133=CARTESIAN_POINT('Origin',(0.,0.,0.));
#10134=CARTESIAN_POINT('',(-0.335465908756113,0.,-1.20190105810224));
#10135=CARTESIAN_POINT('Origin',(-0.379577794185951,0.,-1.1682203282434));
#10136=CARTESIAN_POINT('',(-0.246749348660852,0.,-1.22320001975977));
#10137=CARTESIAN_POINT('Origin',(0.,0.,0.));
#10138=CARTESIAN_POINT('',(-0.143317017690053,0.,-1.23958209161204));
#10139=CARTESIAN_POINT('Origin',(-0.192154639568406,0.,-1.21321664662686));
#10140=CARTESIAN_POINT('',(-0.0523608139934479,0.,-1.24674050008925));
#10141=CARTESIAN_POINT('Origin',(0.,0.,0.));
#10142=CARTESIAN_POINT('',(0.0523608139934481,0.,-1.24674050008925));
#10143=CARTESIAN_POINT('Origin',(7.52141045863017E-17,0.,-1.22833954473516));
#10144=CARTESIAN_POINT('',(0.143317017690053,0.,-1.23958209161204));
#10145=CARTESIAN_POINT('Origin',(0.,0.,0.));
#10146=CARTESIAN_POINT('',(0.246749348660852,0.,-1.22320001975977));
#10147=CARTESIAN_POINT('Origin',(0.192154639568406,0.,-1.21321664662686));
#10148=CARTESIAN_POINT('',(0.335465908756113,0.,-1.20190105810224));
#10149=CARTESIAN_POINT('Origin',(0.,0.,0.));
#10150=CARTESIAN_POINT('',(0.435062095450087,0.,-1.16954029537568));
#10151=CARTESIAN_POINT('Origin',(0.379577794185951,0.,-1.1682203282434));
#10152=CARTESIAN_POINT('',(0.519354515801077,0.,-1.13462523166105));
#10153=CARTESIAN_POINT('Origin',(0.,0.,0.));
#10154=CARTESIAN_POINT('',(0.612662169561028,0.,-1.08708260743774));
#10155=CARTESIAN_POINT('Origin',(0.557654483764164,0.,-1.0944585482776));
#10156=CARTESIAN_POINT('',(0.690454891028201,0.,-1.0394111664111));
#10157=CARTESIAN_POINT('Origin',(0.,0.,0.));
#10158=CARTESIAN_POINT('',(0.775176467748211,0.,-0.977857337884349));
#10159=CARTESIAN_POINT('Origin',(0.721999869202979,0.,-0.993747566553533));
#10160=CARTESIAN_POINT('',(0.844553975349804,0.,-0.918603348636233));
#10161=CARTESIAN_POINT('Origin',(0.,0.,0.));
#10162=CARTESIAN_POINT('',(0.918603348636233,0.,-0.844553975349804));
#10163=CARTESIAN_POINT('Origin',(0.86856722168183,0.,-0.86856722168183));
#10164=CARTESIAN_POINT('',(0.977857337884349,0.,-0.775176467748211));
#10165=CARTESIAN_POINT('Origin',(0.,0.,0.));
#10166=CARTESIAN_POINT('',(1.0394111664111,0.,-0.690454891028201));
#10167=CARTESIAN_POINT('Origin',(0.993747566553533,0.,-0.721999869202979));
#10168=CARTESIAN_POINT('',(1.08708260743774,0.,-0.612662169561028));
#10169=CARTESIAN_POINT('Origin',(0.,0.,0.));
#10170=CARTESIAN_POINT('',(1.13462523166105,0.,-0.519354515801077));
#10171=CARTESIAN_POINT('Origin',(1.0944585482776,0.,-0.557654483764164));
#10172=CARTESIAN_POINT('',(1.16954029537568,0.,-0.43506209545009));
#10173=CARTESIAN_POINT('Origin',(0.,0.,0.));
#10174=CARTESIAN_POINT('',(1.20190105810224,0.,-0.33546590875611));
#10175=CARTESIAN_POINT('Origin',(1.1682203282434,0.,-0.379577794185951));
#10176=CARTESIAN_POINT('',(1.22320001975977,0.,-0.246749348660852));
#10177=CARTESIAN_POINT('Origin',(0.,0.,0.));
#10178=CARTESIAN_POINT('',(1.23958209161204,0.,-0.143317017690053));
#10179=CARTESIAN_POINT('Origin',(1.21321664662686,0.,-0.192154639568406));
#10180=CARTESIAN_POINT('',(1.24674050008925,0.,-0.052360813993451));
#10181=CARTESIAN_POINT('Origin',(0.,0.,0.));
#10182=CARTESIAN_POINT('',(1.24674050008925,0.,0.052360813993451));
#10183=CARTESIAN_POINT('Origin',(1.22833954473516,0.,0.));
#10184=CARTESIAN_POINT('Origin',(0.,0.,0.));
#10185=CARTESIAN_POINT('Origin',(0.,0.,0.));
#10186=CARTESIAN_POINT('',(-1.4,-0.1,1.71450551880629E-16));
#10187=CARTESIAN_POINT('Origin',(0.,-0.1,0.));
#10188=CARTESIAN_POINT('',(-1.4,0.,-1.71450551880629E-16));
#10189=CARTESIAN_POINT('Origin',(0.,-0.1,0.));
#10190=CARTESIAN_POINT('Origin',(0.,0.75,0.));
#10191=CARTESIAN_POINT('',(-1.4,0.75,1.71450551880629E-16));
#10192=CARTESIAN_POINT('Origin',(0.,0.75,0.));
#10193=CARTESIAN_POINT('',(1.22320001975977,0.75,0.246749348660852));
#10194=CARTESIAN_POINT('',(1.23958209161204,0.75,0.143317017690053));
#10195=CARTESIAN_POINT('Origin',(1.21321664662686,0.75,0.192154639568406));
#10196=CARTESIAN_POINT('',(1.24674050008925,0.75,0.052360813993448));
#10197=CARTESIAN_POINT('Origin',(0.,0.75,0.));
#10198=CARTESIAN_POINT('',(1.24674050008925,0.75,-0.052360813993448));
#10199=CARTESIAN_POINT('Origin',(1.22833954473516,0.75,0.));
#10200=CARTESIAN_POINT('',(1.23958209161204,0.75,-0.143317017690053));
#10201=CARTESIAN_POINT('Origin',(0.,0.75,0.));
#10202=CARTESIAN_POINT('',(1.22320001975977,0.75,-0.246749348660852));
#10203=CARTESIAN_POINT('Origin',(1.21321664662686,0.75,-0.192154639568406));
#10204=CARTESIAN_POINT('',(1.20190105810224,0.75,-0.335465908756113));
#10205=CARTESIAN_POINT('Origin',(0.,0.75,0.));
#10206=CARTESIAN_POINT('',(1.16954029537568,0.75,-0.435062095450087));
#10207=CARTESIAN_POINT('Origin',(1.1682203282434,0.75,-0.379577794185951));
#10208=CARTESIAN_POINT('',(1.13462523166105,0.75,-0.519354515801077));
#10209=CARTESIAN_POINT('Origin',(0.,0.75,0.));
#10210=CARTESIAN_POINT('',(1.08708260743774,0.75,-0.612662169561028));
#10211=CARTESIAN_POINT('Origin',(1.0944585482776,0.75,-0.557654483764164));
#10212=CARTESIAN_POINT('',(1.0394111664111,0.75,-0.690454891028201));
#10213=CARTESIAN_POINT('Origin',(0.,0.75,0.));
#10214=CARTESIAN_POINT('',(0.977857337884349,0.75,-0.775176467748211));
#10215=CARTESIAN_POINT('Origin',(0.993747566553533,0.75,-0.721999869202979));
#10216=CARTESIAN_POINT('',(0.918603348636233,0.75,-0.844553975349804));
#10217=CARTESIAN_POINT('Origin',(0.,0.75,0.));
#10218=CARTESIAN_POINT('',(0.844553975349804,0.75,-0.918603348636233));
#10219=CARTESIAN_POINT('Origin',(0.86856722168183,0.75,-0.86856722168183));
#10220=CARTESIAN_POINT('',(0.775176467748211,0.75,-0.977857337884349));
#10221=CARTESIAN_POINT('Origin',(0.,0.75,0.));
#10222=CARTESIAN_POINT('',(0.690454891028201,0.75,-1.0394111664111));
#10223=CARTESIAN_POINT('Origin',(0.721999869202979,0.75,-0.993747566553533));
#10224=CARTESIAN_POINT('',(0.612662169561028,0.75,-1.08708260743774));
#10225=CARTESIAN_POINT('Origin',(0.,0.75,0.));
#10226=CARTESIAN_POINT('',(0.519354515801077,0.75,-1.13462523166105));
#10227=CARTESIAN_POINT('Origin',(0.557654483764164,0.75,-1.0944585482776));
#10228=CARTESIAN_POINT('',(0.435062095450087,0.75,-1.16954029537568));
#10229=CARTESIAN_POINT('Origin',(0.,0.75,0.));
#10230=CARTESIAN_POINT('',(0.335465908756113,0.75,-1.20190105810224));
#10231=CARTESIAN_POINT('Origin',(0.379577794185951,0.75,-1.1682203282434));
#10232=CARTESIAN_POINT('',(0.246749348660852,0.75,-1.22320001975977));
#10233=CARTESIAN_POINT('Origin',(0.,0.75,0.));
#10234=CARTESIAN_POINT('',(0.143317017690053,0.75,-1.23958209161204));
#10235=CARTESIAN_POINT('Origin',(0.192154639568406,0.75,-1.21321664662686));
#10236=CARTESIAN_POINT('',(0.0523608139934481,0.75,-1.24674050008925));
#10237=CARTESIAN_POINT('Origin',(0.,0.75,0.));
#10238=CARTESIAN_POINT('',(-0.0523608139934479,0.75,-1.24674050008925));
#10239=CARTESIAN_POINT('Origin',(7.52141045863017E-17,0.75,-1.22833954473516));
#10240=CARTESIAN_POINT('',(-0.143317017690053,0.75,-1.23958209161204));
#10241=CARTESIAN_POINT('Origin',(0.,0.75,0.));
#10242=CARTESIAN_POINT('',(-0.246749348660852,0.75,-1.22320001975977));
#10243=CARTESIAN_POINT('Origin',(-0.192154639568406,0.75,-1.21321664662686));
#10244=CARTESIAN_POINT('',(-0.335465908756113,0.75,-1.20190105810224));
#10245=CARTESIAN_POINT('Origin',(0.,0.75,0.));
#10246=CARTESIAN_POINT('',(-0.435062095450087,0.75,-1.16954029537568));
#10247=CARTESIAN_POINT('Origin',(-0.379577794185951,0.75,-1.1682203282434));
#10248=CARTESIAN_POINT('',(-0.519354515801077,0.75,-1.13462523166105));
#10249=CARTESIAN_POINT('Origin',(0.,0.75,0.));
#10250=CARTESIAN_POINT('',(-0.612662169561028,0.75,-1.08708260743774));
#10251=CARTESIAN_POINT('Origin',(-0.557654483764164,0.75,-1.0944585482776));
#10252=CARTESIAN_POINT('',(-0.690454891028201,0.75,-1.0394111664111));
#10253=CARTESIAN_POINT('Origin',(0.,0.75,0.));
#10254=CARTESIAN_POINT('',(-0.775176467748211,0.75,-0.977857337884348));
#10255=CARTESIAN_POINT('Origin',(-0.721999869202979,0.75,-0.993747566553533));
#10256=CARTESIAN_POINT('',(-0.844553975349804,0.75,-0.918603348636233));
#10257=CARTESIAN_POINT('Origin',(0.,0.75,0.));
#10258=CARTESIAN_POINT('',(-0.918603348636233,0.75,-0.844553975349804));
#10259=CARTESIAN_POINT('Origin',(-0.86856722168183,0.75,-0.86856722168183));
#10260=CARTESIAN_POINT('',(-0.977857337884349,0.75,-0.775176467748211));
#10261=CARTESIAN_POINT('Origin',(0.,0.75,0.));
#10262=CARTESIAN_POINT('',(-1.0394111664111,0.75,-0.690454891028201));
#10263=CARTESIAN_POINT('Origin',(-0.993747566553533,0.75,-0.721999869202979));
#10264=CARTESIAN_POINT('',(-1.08708260743774,0.75,-0.612662169561029));
#10265=CARTESIAN_POINT('Origin',(0.,0.75,0.));
#10266=CARTESIAN_POINT('',(-1.13462523166105,0.75,-0.519354515801077));
#10267=CARTESIAN_POINT('Origin',(-1.0944585482776,0.75,-0.557654483764164));
#10268=CARTESIAN_POINT('',(-1.16954029537568,0.75,-0.435062095450087));
#10269=CARTESIAN_POINT('Origin',(0.,0.75,0.));
#10270=CARTESIAN_POINT('',(-1.20190105810224,0.75,-0.335465908756113));
#10271=CARTESIAN_POINT('Origin',(-1.1682203282434,0.75,-0.379577794185951));
#10272=CARTESIAN_POINT('',(-1.22320001975977,0.75,-0.246749348660852));
#10273=CARTESIAN_POINT('Origin',(0.,0.75,0.));
#10274=CARTESIAN_POINT('',(-1.23958209161204,0.75,-0.143317017690053));
#10275=CARTESIAN_POINT('Origin',(-1.21321664662686,0.75,-0.192154639568406));
#10276=CARTESIAN_POINT('',(-1.24674050008925,0.75,-0.0523608139934482));
#10277=CARTESIAN_POINT('Origin',(0.,0.75,0.));
#10278=CARTESIAN_POINT('',(-1.24674050008925,0.75,0.0523608139934479));
#10279=CARTESIAN_POINT('Origin',(-1.22833954473516,0.75,-1.50428209172603E-16));
#10280=CARTESIAN_POINT('',(-1.23958209161204,0.75,0.143317017690053));
#10281=CARTESIAN_POINT('Origin',(0.,0.75,0.));
#10282=CARTESIAN_POINT('',(-1.22320001975977,0.75,0.246749348660851));
#10283=CARTESIAN_POINT('Origin',(-1.21321664662686,0.75,0.192154639568406));
#10284=CARTESIAN_POINT('',(-1.20190105810224,0.75,0.335465908756113));
#10285=CARTESIAN_POINT('Origin',(0.,0.75,0.));
#10286=CARTESIAN_POINT('',(-1.16954029537568,0.75,0.435062095450087));
#10287=CARTESIAN_POINT('Origin',(-1.1682203282434,0.75,0.379577794185951));
#10288=CARTESIAN_POINT('',(-1.13462523166105,0.75,0.519354515801077));
#10289=CARTESIAN_POINT('Origin',(0.,0.75,0.));
#10290=CARTESIAN_POINT('',(-1.08708260743774,0.75,0.612662169561028));
#10291=CARTESIAN_POINT('Origin',(-1.0944585482776,0.75,0.557654483764164));
#10292=CARTESIAN_POINT('',(-1.0394111664111,0.75,0.690454891028201));
#10293=CARTESIAN_POINT('Origin',(0.,0.75,0.));
#10294=CARTESIAN_POINT('',(-0.977857337884348,0.75,0.775176467748211));
#10295=CARTESIAN_POINT('Origin',(-0.993747566553533,0.75,0.721999869202979));
#10296=CARTESIAN_POINT('',(-0.918603348636233,0.75,0.844553975349804));
#10297=CARTESIAN_POINT('Origin',(0.,0.75,0.));
#10298=CARTESIAN_POINT('',(-0.844553975349804,0.75,0.918603348636233));
#10299=CARTESIAN_POINT('Origin',(-0.86856722168183,0.75,0.86856722168183));
#10300=CARTESIAN_POINT('',(-0.775176467748211,0.75,0.977857337884349));
#10301=CARTESIAN_POINT('Origin',(0.,0.75,0.));
#10302=CARTESIAN_POINT('',(-0.690454891028201,0.75,1.0394111664111));
#10303=CARTESIAN_POINT('Origin',(-0.721999869202979,0.75,0.993747566553533));
#10304=CARTESIAN_POINT('',(-0.612662169561029,0.75,1.08708260743774));
#10305=CARTESIAN_POINT('Origin',(0.,0.75,0.));
#10306=CARTESIAN_POINT('',(-0.519354515801077,0.75,1.13462523166105));
#10307=CARTESIAN_POINT('Origin',(-0.557654483764164,0.75,1.0944585482776));
#10308=CARTESIAN_POINT('',(-0.435062095450087,0.75,1.16954029537568));
#10309=CARTESIAN_POINT('Origin',(0.,0.75,0.));
#10310=CARTESIAN_POINT('',(-0.335465908756113,0.75,1.20190105810224));
#10311=CARTESIAN_POINT('Origin',(-0.379577794185951,0.75,1.1682203282434));
#10312=CARTESIAN_POINT('',(-0.246749348660852,0.75,1.22320001975977));
#10313=CARTESIAN_POINT('Origin',(0.,0.75,0.));
#10314=CARTESIAN_POINT('',(-0.143317017690053,0.75,1.23958209161204));
#10315=CARTESIAN_POINT('Origin',(-0.192154639568406,0.75,1.21321664662686));
#10316=CARTESIAN_POINT('',(-0.0523608139934483,0.75,1.24674050008925));
#10317=CARTESIAN_POINT('Origin',(0.,0.75,0.));
#10318=CARTESIAN_POINT('',(0.0523608139934478,0.75,1.24674050008925));
#10319=CARTESIAN_POINT('Origin',(-2.25642313758905E-16,0.75,1.22833954473516));
#10320=CARTESIAN_POINT('',(0.143317017690053,0.75,1.23958209161204));
#10321=CARTESIAN_POINT('Origin',(0.,0.75,0.));
#10322=CARTESIAN_POINT('',(0.246749348660851,0.75,1.22320001975977));
#10323=CARTESIAN_POINT('Origin',(0.192154639568406,0.75,1.21321664662686));
#10324=CARTESIAN_POINT('',(0.335465908756113,0.75,1.20190105810224));
#10325=CARTESIAN_POINT('Origin',(0.,0.75,0.));
#10326=CARTESIAN_POINT('',(0.435062095450087,0.75,1.16954029537568));
#10327=CARTESIAN_POINT('Origin',(0.379577794185951,0.75,1.1682203282434));
#10328=CARTESIAN_POINT('',(0.519354515801077,0.75,1.13462523166105));
#10329=CARTESIAN_POINT('Origin',(0.,0.75,0.));
#10330=CARTESIAN_POINT('',(0.612662169561028,0.75,1.08708260743774));
#10331=CARTESIAN_POINT('Origin',(0.557654483764164,0.75,1.0944585482776));
#10332=CARTESIAN_POINT('',(0.690454891028201,0.75,1.0394111664111));
#10333=CARTESIAN_POINT('Origin',(0.,0.75,0.));
#10334=CARTESIAN_POINT('',(0.775176467748211,0.75,0.977857337884349));
#10335=CARTESIAN_POINT('Origin',(0.721999869202979,0.75,0.993747566553533));
#10336=CARTESIAN_POINT('',(0.844553975349804,0.75,0.918603348636233));
#10337=CARTESIAN_POINT('Origin',(0.,0.75,0.));
#10338=CARTESIAN_POINT('',(0.918603348636233,0.75,0.844553975349804));
#10339=CARTESIAN_POINT('Origin',(0.86856722168183,0.75,0.86856722168183));
#10340=CARTESIAN_POINT('',(0.977857337884349,0.75,0.775176467748211));
#10341=CARTESIAN_POINT('Origin',(0.,0.75,0.));
#10342=CARTESIAN_POINT('',(1.0394111664111,0.75,0.690454891028201));
#10343=CARTESIAN_POINT('Origin',(0.993747566553533,0.75,0.72199986920298));
#10344=CARTESIAN_POINT('',(1.08708260743774,0.75,0.612662169561029));
#10345=CARTESIAN_POINT('Origin',(0.,0.75,0.));
#10346=CARTESIAN_POINT('',(1.13462523166105,0.75,0.519354515801077));
#10347=CARTESIAN_POINT('Origin',(1.0944585482776,0.75,0.557654483764164));
#10348=CARTESIAN_POINT('',(1.16954029537568,0.75,0.435062095450087));
#10349=CARTESIAN_POINT('Origin',(0.,0.75,0.));
#10350=CARTESIAN_POINT('',(1.20190105810224,0.75,0.335465908756113));
#10351=CARTESIAN_POINT('Origin',(1.1682203282434,0.75,0.379577794185952));
#10352=CARTESIAN_POINT('Origin',(0.,0.75,0.));
#10353=CARTESIAN_POINT('Origin',(0.,0.75,0.));
#10354=CARTESIAN_POINT('',(-1.4,0.75,1.71450551880629E-16));
#10355=CARTESIAN_POINT('Origin',(1.21321664662686,0.,0.192154639568406));
#10356=CARTESIAN_POINT('',(1.23958209161204,0.,0.14331701769005));
#10357=CARTESIAN_POINT('',(1.22320001975977,0.,0.246749348660855));
#10358=CARTESIAN_POINT('Origin',(0.,0.,0.));
#10359=CARTESIAN_POINT('',(1.20190105810224,0.,0.33546590875611));
#10360=CARTESIAN_POINT('Origin',(1.1682203282434,0.,0.379577794185952));
#10361=CARTESIAN_POINT('',(1.16954029537568,0.,0.43506209545009));
#10362=CARTESIAN_POINT('Origin',(0.,0.,0.));
#10363=CARTESIAN_POINT('',(1.13462523166105,0.,0.519354515801074));
#10364=CARTESIAN_POINT('Origin',(1.0944585482776,0.,0.557654483764164));
#10365=CARTESIAN_POINT('',(1.08708260743774,0.,0.612662169561031));
#10366=CARTESIAN_POINT('Origin',(0.,0.,0.));
#10367=CARTESIAN_POINT('',(1.03941116641111,0.,0.690454891028199));
#10368=CARTESIAN_POINT('Origin',(0.993747566553533,0.,0.72199986920298));
#10369=CARTESIAN_POINT('',(0.977857337884347,0.,0.775176467748214));
#10370=CARTESIAN_POINT('Origin',(0.,0.,0.));
#10371=CARTESIAN_POINT('',(0.918603348636235,0.,0.844553975349802));
#10372=CARTESIAN_POINT('Origin',(0.86856722168183,0.,0.86856722168183));
#10373=CARTESIAN_POINT('',(0.844553975349802,0.,0.918603348636235));
#10374=CARTESIAN_POINT('Origin',(0.,0.,0.));
#10375=CARTESIAN_POINT('',(0.775176467748213,0.,0.977857337884347));
#10376=CARTESIAN_POINT('Origin',(0.721999869202979,0.,0.993747566553533));
#10377=CARTESIAN_POINT('',(0.690454891028198,0.,1.03941116641111));
#10378=CARTESIAN_POINT('Origin',(0.,0.,0.));
#10379=CARTESIAN_POINT('',(0.612662169561031,0.,1.08708260743774));
#10380=CARTESIAN_POINT('Origin',(0.557654483764164,0.,1.0944585482776));
#10381=CARTESIAN_POINT('',(0.519354515801074,0.,1.13462523166105));
#10382=CARTESIAN_POINT('Origin',(0.,0.,0.));
#10383=CARTESIAN_POINT('',(0.43506209545009,0.,1.16954029537568));
#10384=CARTESIAN_POINT('Origin',(0.379577794185951,0.,1.1682203282434));
#10385=CARTESIAN_POINT('',(0.33546590875611,0.,1.20190105810224));
#10386=CARTESIAN_POINT('Origin',(0.,0.,0.));
#10387=CARTESIAN_POINT('',(0.246749348660854,0.,1.22320001975977));
#10388=CARTESIAN_POINT('Origin',(0.192154639568406,0.,1.21321664662686));
#10389=CARTESIAN_POINT('',(0.14331701769005,0.,1.23958209161204));
#10390=CARTESIAN_POINT('Origin',(0.,0.,0.));
#10391=CARTESIAN_POINT('',(0.0523608139934508,0.,1.24674050008925));
#10392=CARTESIAN_POINT('Origin',(-2.25642313758905E-16,0.,1.22833954473516));
#10393=CARTESIAN_POINT('',(-0.0523608139934513,0.,1.24674050008925));
#10394=CARTESIAN_POINT('Origin',(0.,0.,0.));
#10395=CARTESIAN_POINT('',(-0.14331701769005,0.,1.23958209161204));
#10396=CARTESIAN_POINT('Origin',(-0.192154639568406,0.,1.21321664662686));
#10397=CARTESIAN_POINT('',(-0.246749348660855,0.,1.22320001975977));
#10398=CARTESIAN_POINT('Origin',(0.,0.,0.));
#10399=CARTESIAN_POINT('',(-0.33546590875611,0.,1.20190105810224));
#10400=CARTESIAN_POINT('Origin',(-0.379577794185951,0.,1.1682203282434));
#10401=CARTESIAN_POINT('',(-0.43506209545009,0.,1.16954029537568));
#10402=CARTESIAN_POINT('Origin',(0.,0.,0.));
#10403=CARTESIAN_POINT('',(-0.519354515801074,0.,1.13462523166105));
#10404=CARTESIAN_POINT('Origin',(-0.557654483764164,0.,1.0944585482776));
#10405=CARTESIAN_POINT('',(-0.612662169561031,0.,1.08708260743774));
#10406=CARTESIAN_POINT('Origin',(0.,0.,0.));
#10407=CARTESIAN_POINT('',(-0.690454891028199,0.,1.03941116641111));
#10408=CARTESIAN_POINT('Origin',(-0.721999869202979,0.,0.993747566553533));
#10409=CARTESIAN_POINT('',(-0.775176467748213,0.,0.977857337884347));
#10410=CARTESIAN_POINT('Origin',(0.,0.,0.));
#10411=CARTESIAN_POINT('',(-0.844553975349802,0.,0.918603348636235));
#10412=CARTESIAN_POINT('Origin',(-0.86856722168183,0.,0.86856722168183));
#10413=CARTESIAN_POINT('',(-0.918603348636235,0.,0.844553975349802));
#10414=CARTESIAN_POINT('Origin',(0.,0.,0.));
#10415=CARTESIAN_POINT('',(-0.977857337884347,0.,0.775176467748213));
#10416=CARTESIAN_POINT('Origin',(-0.993747566553533,0.,0.721999869202979));
#10417=CARTESIAN_POINT('',(-1.03941116641111,0.,0.690454891028198));
#10418=CARTESIAN_POINT('Origin',(0.,0.,0.));
#10419=CARTESIAN_POINT('',(-1.08708260743774,0.,0.612662169561031));
#10420=CARTESIAN_POINT('Origin',(-1.0944585482776,0.,0.557654483764164));
#10421=CARTESIAN_POINT('',(-1.13462523166105,0.,0.519354515801074));
#10422=CARTESIAN_POINT('Origin',(0.,0.,0.));
#10423=CARTESIAN_POINT('',(-1.16954029537568,0.,0.43506209545009));
#10424=CARTESIAN_POINT('Origin',(-1.1682203282434,0.,0.379577794185951));
#10425=CARTESIAN_POINT('',(-1.20190105810224,0.,0.33546590875611));
#10426=CARTESIAN_POINT('Origin',(0.,0.,0.));
#10427=CARTESIAN_POINT('',(-1.22320001975977,0.,0.246749348660854));
#10428=CARTESIAN_POINT('Origin',(-1.21321664662686,0.,0.192154639568406));
#10429=CARTESIAN_POINT('',(-1.23958209161204,0.,0.14331701769005));
#10430=CARTESIAN_POINT('Origin',(0.,0.,0.));
#10431=CARTESIAN_POINT('',(-1.24674050008925,0.,0.0523608139934509));
#10432=CARTESIAN_POINT('Origin',(-1.22833954473516,0.,-1.50428209172603E-16));
#10433=CARTESIAN_POINT('',(-1.24674050008925,0.,-0.0523608139934512));
#10434=CARTESIAN_POINT('Origin',(0.,0.,0.));
#10435=CARTESIAN_POINT('',(-1.23958209161204,0.,-0.14331701769005));
#10436=CARTESIAN_POINT('Origin',(-1.21321664662686,0.,-0.192154639568406));
#10437=CARTESIAN_POINT('',(-1.22320001975977,0.,-0.246749348660855));
#10438=CARTESIAN_POINT('Origin',(0.,0.,0.));
#10439=CARTESIAN_POINT('',(-1.20190105810224,0.,-0.33546590875611));
#10440=CARTESIAN_POINT('Origin',(-1.1682203282434,0.,-0.379577794185951));
#10441=CARTESIAN_POINT('',(-1.16954029537568,0.,-0.43506209545009));
#10442=CARTESIAN_POINT('Origin',(0.,0.,0.));
#10443=CARTESIAN_POINT('',(-1.13462523166105,0.,-0.519354515801074));
#10444=CARTESIAN_POINT('Origin',(-1.0944585482776,0.,-0.557654483764164));
#10445=CARTESIAN_POINT('',(-1.08708260743774,0.,-0.612662169561031));
#10446=CARTESIAN_POINT('Origin',(0.,0.,0.));
#10447=CARTESIAN_POINT('',(-1.03941116641111,0.,-0.690454891028199));
#10448=CARTESIAN_POINT('Origin',(-0.993747566553533,0.,-0.721999869202979));
#10449=CARTESIAN_POINT('',(-0.977857337884347,0.,-0.775176467748213));
#10450=CARTESIAN_POINT('Origin',(0.,0.,0.));
#10451=CARTESIAN_POINT('',(-0.918603348636235,0.,-0.844553975349802));
#10452=CARTESIAN_POINT('Origin',(-0.86856722168183,0.,-0.86856722168183));
#10453=CARTESIAN_POINT('',(-0.844553975349802,0.,-0.918603348636235));
#10454=CARTESIAN_POINT('Origin',(0.,0.,0.));
#10455=CARTESIAN_POINT('',(-0.775176467748213,0.,-0.977857337884347));
#10456=CARTESIAN_POINT('Origin',(-0.721999869202979,0.,-0.993747566553533));
#10457=CARTESIAN_POINT('',(-0.690454891028198,0.,-1.03941116641111));
#10458=CARTESIAN_POINT('Origin',(0.,0.,0.));
#10459=CARTESIAN_POINT('',(-0.612662169561031,0.,-1.08708260743774));
#10460=CARTESIAN_POINT('Origin',(-0.557654483764164,0.,-1.0944585482776));
#10461=CARTESIAN_POINT('',(-0.519354515801074,0.,-1.13462523166105));
#10462=CARTESIAN_POINT('Origin',(0.,0.,0.));
#10463=CARTESIAN_POINT('',(-0.43506209545009,0.,-1.16954029537568));
#10464=CARTESIAN_POINT('Origin',(-0.379577794185951,0.,-1.1682203282434));
#10465=CARTESIAN_POINT('',(-0.33546590875611,0.,-1.20190105810224));
#10466=CARTESIAN_POINT('Origin',(0.,0.,0.));
#10467=CARTESIAN_POINT('',(-0.246749348660854,0.,-1.22320001975977));
#10468=CARTESIAN_POINT('Origin',(-0.192154639568406,0.,-1.21321664662686));
#10469=CARTESIAN_POINT('',(-0.14331701769005,0.,-1.23958209161204));
#10470=CARTESIAN_POINT('Origin',(0.,0.,0.));
#10471=CARTESIAN_POINT('',(-0.052360813993451,0.,-1.24674050008925));
#10472=CARTESIAN_POINT('Origin',(7.52141045863017E-17,0.,-1.22833954473516));
#10473=CARTESIAN_POINT('',(0.0523608139934511,0.,-1.24674050008925));
#10474=CARTESIAN_POINT('Origin',(0.,0.,0.));
#10475=CARTESIAN_POINT('',(0.14331701769005,0.,-1.23958209161204));
#10476=CARTESIAN_POINT('Origin',(0.192154639568406,0.,-1.21321664662686));
#10477=CARTESIAN_POINT('',(0.246749348660855,0.,-1.22320001975977));
#10478=CARTESIAN_POINT('Origin',(0.,0.,0.));
#10479=CARTESIAN_POINT('',(0.33546590875611,0.,-1.20190105810224));
#10480=CARTESIAN_POINT('Origin',(0.379577794185951,0.,-1.1682203282434));
#10481=CARTESIAN_POINT('',(0.43506209545009,0.,-1.16954029537568));
#10482=CARTESIAN_POINT('Origin',(0.,0.,0.));
#10483=CARTESIAN_POINT('',(0.519354515801074,0.,-1.13462523166105));
#10484=CARTESIAN_POINT('Origin',(0.557654483764164,0.,-1.0944585482776));
#10485=CARTESIAN_POINT('',(0.612662169561031,0.,-1.08708260743774));
#10486=CARTESIAN_POINT('Origin',(0.,0.,0.));
#10487=CARTESIAN_POINT('',(0.690454891028198,0.,-1.03941116641111));
#10488=CARTESIAN_POINT('Origin',(0.721999869202979,0.,-0.993747566553533));
#10489=CARTESIAN_POINT('',(0.775176467748213,0.,-0.977857337884347));
#10490=CARTESIAN_POINT('Origin',(0.,0.,0.));
#10491=CARTESIAN_POINT('',(0.844553975349802,0.,-0.918603348636235));
#10492=CARTESIAN_POINT('Origin',(0.86856722168183,0.,-0.86856722168183));
#10493=CARTESIAN_POINT('',(0.918603348636235,0.,-0.844553975349802));
#10494=CARTESIAN_POINT('Origin',(0.,0.,0.));
#10495=CARTESIAN_POINT('',(0.977857337884347,0.,-0.775176467748213));
#10496=CARTESIAN_POINT('Origin',(0.993747566553533,0.,-0.721999869202979));
#10497=CARTESIAN_POINT('',(1.03941116641111,0.,-0.690454891028198));
#10498=CARTESIAN_POINT('Origin',(0.,0.,0.));
#10499=CARTESIAN_POINT('',(1.08708260743774,0.,-0.612662169561031));
#10500=CARTESIAN_POINT('Origin',(1.0944585482776,0.,-0.557654483764164));
#10501=CARTESIAN_POINT('',(1.13462523166105,0.,-0.519354515801074));
#10502=CARTESIAN_POINT('Origin',(0.,0.,0.));
#10503=CARTESIAN_POINT('',(1.16954029537568,0.,-0.43506209545009));
#10504=CARTESIAN_POINT('Origin',(1.1682203282434,0.,-0.379577794185951));
#10505=CARTESIAN_POINT('',(1.20190105810224,0.,-0.33546590875611));
#10506=CARTESIAN_POINT('Origin',(0.,0.,0.));
#10507=CARTESIAN_POINT('',(1.22320001975977,0.,-0.246749348660855));
#10508=CARTESIAN_POINT('Origin',(1.21321664662686,0.,-0.192154639568406));
#10509=CARTESIAN_POINT('',(1.23958209161204,0.,-0.14331701769005));
#10510=CARTESIAN_POINT('Origin',(0.,0.,0.));
#10511=CARTESIAN_POINT('',(1.24674050008925,0.,0.052360813993451));
#10512=CARTESIAN_POINT('Origin',(1.22833954473516,0.,0.));
#10513=CARTESIAN_POINT('',(1.24674050008925,0.,-0.052360813993451));
#10514=CARTESIAN_POINT('Origin',(0.,0.,0.));
#10786=UNCERTAINTY_MEASURE_WITH_UNIT(LENGTH_MEASURE(0.001),#10822,
'DISTANCE_ACCURACY_VALUE',
'Maximum model space distance between geometric entities at asserted c
onnectivities');
#10791=UNCERTAINTY_MEASURE_WITH_UNIT(LENGTH_MEASURE(0.001),#10822,
'DISTANCE_ACCURACY_VALUE',
'Maximum model space distance between geometric entities at asserted c
onnectivities');
#10816=(
GEOMETRIC_REPRESENTATION_CONTEXT(3)
GLOBAL_UNCERTAINTY_ASSIGNED_CONTEXT((#10786))
GLOBAL_UNIT_ASSIGNED_CONTEXT((#10822,#10824,#10825))
REPRESENTATION_CONTEXT('','3D')
);
#10821=(
GEOMETRIC_REPRESENTATION_CONTEXT(3)
GLOBAL_UNCERTAINTY_ASSIGNED_CONTEXT((#10791))
GLOBAL_UNIT_ASSIGNED_CONTEXT((#10822,#10824,#10825))
REPRESENTATION_CONTEXT('','3D')
);
#10822=(
LENGTH_UNIT()
NAMED_UNIT(*)
SI_UNIT(.CENTI.,.METRE.)
);
#10824=(
NAMED_UNIT(*)
PLANE_ANGLE_UNIT()
SI_UNIT($,.RADIAN.)
);
#10825=(
NAMED_UNIT(*)
SI_UNIT($,.STERADIAN.)
SOLID_ANGLE_UNIT()
);
#10850=SHAPE_DEFINITION_REPRESENTATION(#10898,#10948);
#10898=PRODUCT_DEFINITION_SHAPE('',$,#10978);
#10948=SHAPE_REPRESENTATION('',(#6207),#10816);
#10953=PRODUCT_DEFINITION_CONTEXT('part definition',#11042,'design');
#10978=PRODUCT_DEFINITION(
'Timing Pulley - 2 mm Pitch, 40 Teeth, 12 mm Bore',
'Timing Pulley - 2 mm Pitch, 40 Teeth, 12 mm Bore',#11007,#10953);
#11007=PRODUCT_DEFINITION_FORMATION('',$,#11068);
#11042=APPLICATION_CONTEXT(
'Core Data for Automotive Mechanical Design Process');
#11043=PRODUCT_CONTEXT('part definition',#11042,'mechanical');
#11068=PRODUCT('Timing Pulley - 2 mm Pitch, 40 Teeth, 12 mm Bore',
'Timing Pulley - 2 mm Pitch, 40 Teeth, 12 mm Bore',
'Timing Pulley - 2 mm Pitch, 40 Teeth, 12 mm Bore',(#11043));
#11122=COLOUR_RGB('Sky Blue',0.24,0.69,0.87);
#11123=FILL_AREA_STYLE_COLOUR('',#11122);
#11124=FILL_AREA_STYLE('',(#11123));
#11125=SURFACE_STYLE_FILL_AREA(#11124);
#11126=SURFACE_SIDE_STYLE('',(#11125));
#11127=SURFACE_STYLE_USAGE(.BOTH.,#11126);
#11128=PRESENTATION_STYLE_ASSIGNMENT((#11127));
ENDSEC;
END-ISO-10303-21;
